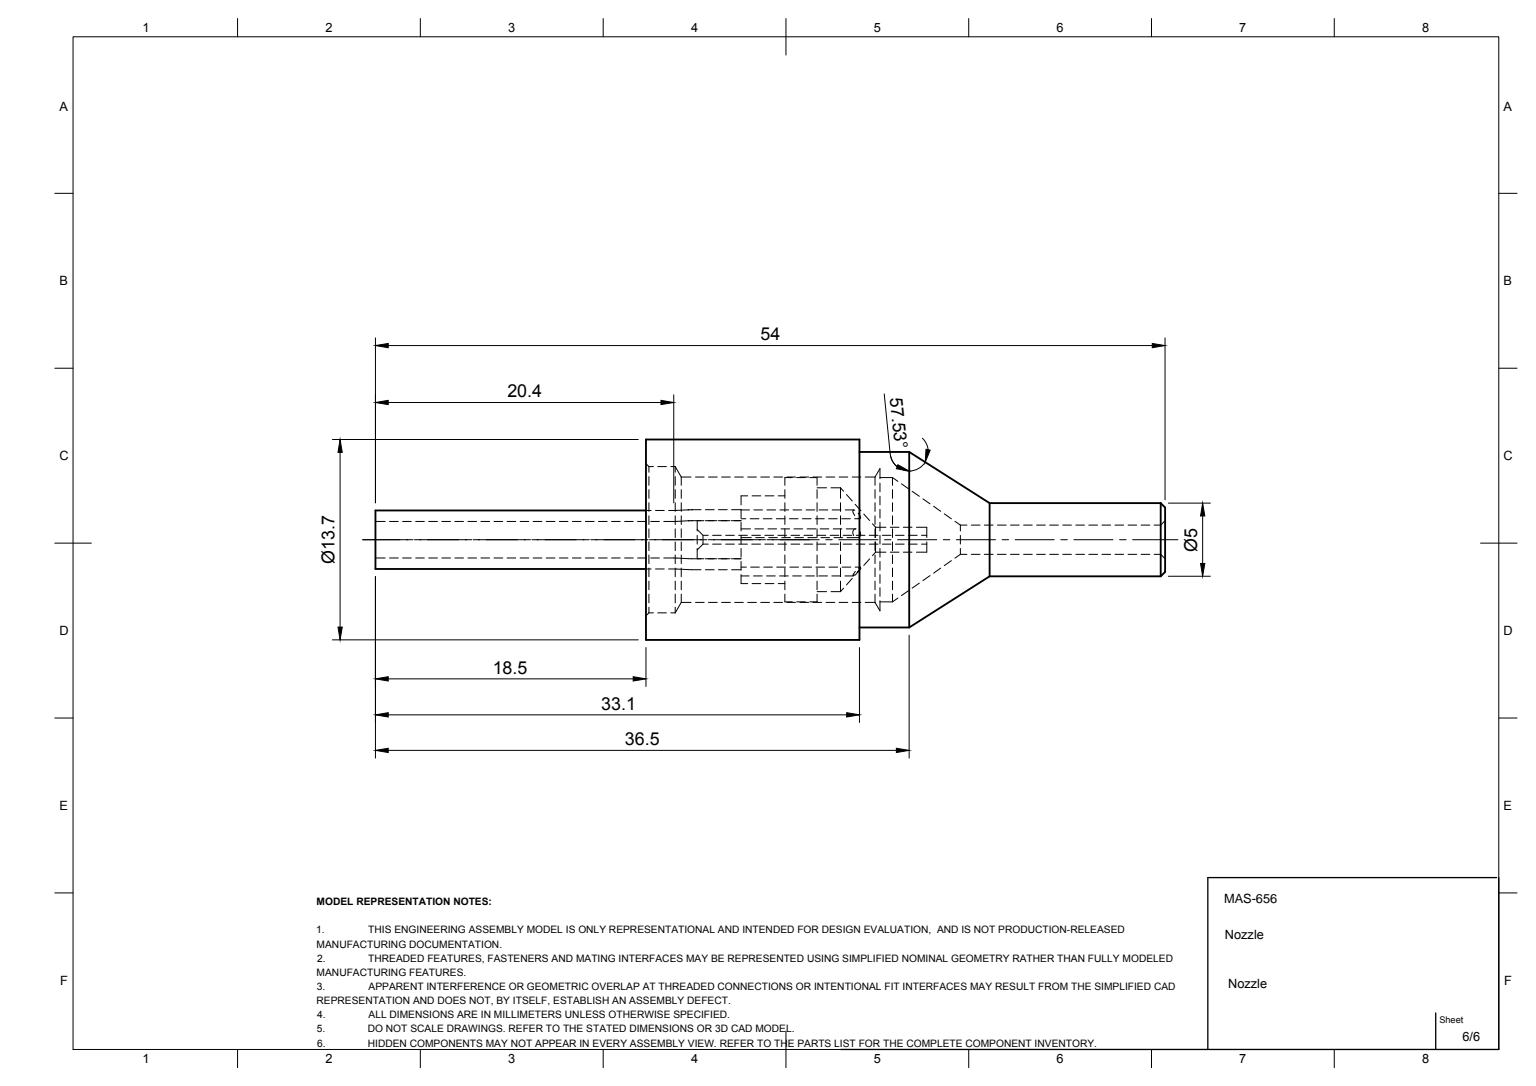
ISO-10303-21;
HEADER;
FILE_DESCRIPTION((''),'2;1');
FILE_NAME('Nozzle.step','2026-10-09T09:41:22-07:00',(''),(''),'','','');
FILE_SCHEMA (('AUTOMOTIVE_DESIGN { 1 0 10303 214 3 1 1 }'));
ENDSEC;
DATA;
#10=MECHANICAL_DESIGN_GEOMETRIC_PRESENTATION_REPRESENTATION('',(#75,#76,#77),#4304);
#55=B_SPLINE_SURFACE_WITH_KNOTS('',5,4,((#3896,#3897,#3898,#3899,#3900),
(#3901,#3902,#3903,#3904,#3905),(#3906,#3907,#3908,#3909,#3910),(#3911,
#3912,#3913,#3914,#3915),(#3916,#3917,#3918,#3919,#3920),(#3921,#3922,#3923,
#3924,#3925),(#3926,#3927,#3928,#3929,#3930),(#3931,#3932,#3933,#3934,#3935),
(#3936,#3937,#3938,#3939,#3940)),.UNSPECIFIED.,.F.,.F.,.F.,(6,3,6),(5,5),
(0.,2.00592385339,5.72401149719),(0.,4.),.UNSPECIFIED.) ;
#56=B_SPLINE_SURFACE_WITH_KNOTS('',5,4,((#4027,#4028,#4029,#4030,#4031),
(#4032,#4033,#4034,#4035,#4036),(#4037,#4038,#4039,#4040,#4041),(#4042,
#4043,#4044,#4045,#4046),(#4047,#4048,#4049,#4050,#4051),(#4052,#4053,#4054,
#4055,#4056),(#4057,#4058,#4059,#4060,#4061),(#4062,#4063,#4064,#4065,#4066),
(#4067,#4068,#4069,#4070,#4071)),.UNSPECIFIED.,.F.,.F.,.F.,(6,3,6),(5,5),
(1.14412490986064,4.56688370431,6.86913676329339),(0.,4.0003840073707),
 .UNSPECIFIED.) ;
#57=B_SPLINE_SURFACE_WITH_KNOTS('',5,4,((#4097,#4098,#4099,#4100,#4101),
(#4102,#4103,#4104,#4105,#4106),(#4107,#4108,#4109,#4110,#4111),(#4112,
#4113,#4114,#4115,#4116),(#4117,#4118,#4119,#4120,#4121),(#4122,#4123,#4124,
#4125,#4126),(#4127,#4128,#4129,#4130,#4131),(#4132,#4133,#4134,#4135,#4136),
(#4137,#4138,#4139,#4140,#4141)),.UNSPECIFIED.,.F.,.F.,.F.,(6,3,6),(5,5),
(1.81018607984298,7.54013629429,10.8709669414987),(-0.00161299974885553,
4.75),.UNSPECIFIED.) ;
#58=B_SPLINE_SURFACE_WITH_KNOTS('',5,4,((#4144,#4145,#4146,#4147,#4148),
(#4149,#4150,#4151,#4152,#4153),(#4154,#4155,#4156,#4157,#4158),(#4159,
#4160,#4161,#4162,#4163),(#4164,#4165,#4166,#4167,#4168),(#4169,#4170,#4171,
#4172,#4173),(#4174,#4175,#4176,#4177,#4178),(#4179,#4180,#4181,#4182,#4183),
(#4184,#4185,#4186,#4187,#4188)),.UNSPECIFIED.,.F.,.F.,.F.,(6,3,6),(5,5),
(-0.00098737241999752,3.59707184609,9.05850997001312),(-0.000987383514799894,
4.75),.UNSPECIFIED.) ;
#59=B_SPLINE_CURVE_WITH_KNOTS('',3,(#3693,#3694,#3695,#3696,#3697,#3698,
#3699,#3700,#3701,#3702,#3703,#3704,#3705,#3706,#3707,#3708,#3709,#3710,
#3711,#3712,#3713,#3714,#3715,#3716,#3717,#3718,#3719,#3720,#3721,#3722,
#3723,#3724,#3725,#3726,#3727,#3728,#3729,#3730),.UNSPECIFIED.,.T.,.F.,
(4,2,2,2,2,2,2,2,2,2,2,2,2,2,2,2,2,2,4),(-0.21266959393403,-0.197090411624007,
-0.181511229313983,-0.168315271544833,-0.161717292660258,-0.155119313775684,
-0.14852133489111,-0.141923356006537,-0.128727398237391,-0.113148215927359,
-0.0975690336173277,-0.0833467314908787,-0.0691244293644297,-0.058954473086547,
-0.0487845168086643,-0.0386145605307833,-0.0284446042529024,-0.0142223021264512,
0.),.UNSPECIFIED.) ;
#60=B_SPLINE_CURVE_WITH_KNOTS('',3,(#3784,#3785,#3786,#3787,#3788,#3789,
#3790,#3791,#3792,#3793,#3794,#3795,#3796,#3797,#3798,#3799,#3800,#3801,
#3802,#3803,#3804,#3805),.UNSPECIFIED.,.F.,.F.,(4,2,2,2,2,2,2,2,2,2,4),
(-0.189267865923668,-0.181511229313965,-0.168315271544809,-0.16171729266023,
-0.155119313775652,-0.148521334891079,-0.141923356006506,-0.128727398237361,
-0.113148215927333,-0.0975690336173056,-0.0836220155565862),
 .UNSPECIFIED.) ;
#61=B_SPLINE_CURVE_WITH_KNOTS('',3,(#3806,#3807,#3808,#3809,#3810,#3811,
#3812,#3813,#3814,#3815,#3816,#3817,#3818,#3819,#3820,#3821,#3822,#3823,
#3824,#3825,#3826,#3827,#3828),.UNSPECIFIED.,.F.,.F.,(4,2,2,2,2,2,2,2,3,
2,4),(-0.0836220155565862,-0.0833467314908613,-0.069124429364417,-0.0589544730865346,
-0.0487845168086522,-0.0386145605307738,-0.0284446042528953,-0.0142223021264476,
0.,0.0155791823100317,0.0234017280103608),.UNSPECIFIED.) ;
#62=B_SPLINE_CURVE_WITH_KNOTS('',3,(#3831,#3832,#3833,#3834,#3835,#3836,
#3837,#3838,#3839,#3840,#3841,#3842,#3843,#3844,#3845,#3846,#3847,#3848,
#3849,#3850,#3851,#3852),.UNSPECIFIED.,.F.,.F.,(4,2,2,2,2,2,2,2,2,2,4),
(-0.189267865923044,-0.181511229313986,-0.16831527154483,-0.161717292660252,
-0.155119313775674,-0.148521334891098,-0.141923356006522,-0.128727398237371,
-0.113148215927341,-0.0975690336173107,-0.083622015556521),
 .UNSPECIFIED.) ;
#63=B_SPLINE_CURVE_WITH_KNOTS('',3,(#3853,#3854,#3855,#3856,#3857,#3858,
#3859,#3860,#3861,#3862,#3863,#3864,#3865,#3866,#3867,#3868,#3869,#3870,
#3871,#3872,#3873,#3874,#3875),.UNSPECIFIED.,.F.,.F.,(4,2,2,2,2,2,2,2,3,
2,4),(-0.083622015556521,-0.0833467314908633,-0.0691244293644159,-0.0589544730865369,
-0.0487845168086579,-0.0386145605307766,-0.0284446042528953,-0.0142223021264477,
0.,0.0155791823100287,0.0234017280109999),.UNSPECIFIED.) ;
#64=B_SPLINE_CURVE_WITH_KNOTS('',3,(#3943,#3944,#3945,#3946,#3947,#3948,
#3949,#3950,#3951,#3952,#3953,#3954,#3955,#3956,#3957,#3958,#3959,#3960,
#3961,#3962,#3963,#3964,#3965,#3966,#3967,#3968,#3969,#3970,#3971,#3972,
#3973,#3974,#3975,#3976,#3977,#3978,#3979,#3980,#3981,#3982,#3983,#3984,
#3985,#3986,#3987,#3988,#3989,#3990,#3991,#3992,#3993,#3994,#3995,#3996,
#3997,#3998,#3999,#4000,#4001,#4002,#4003,#4004,#4005,#4006,#4007,#4008,
#4009,#4010,#4011,#4012,#4013,#4014,#4015,#4016,#4017,#4018,#4019,#4020,
#4021,#4022,#4023,#4024),.UNSPECIFIED.,.F.,.F.,(4,3,3,3,3,3,3,3,3,3,3,3,
3,3,3,3,3,3,3,3,3,3,3,3,3,3,3,4),(0.,0.225460129220956,0.453336599536279,
0.681938236445323,0.91060483211705,1.13866755087004,1.36461264231086,1.58819548811847,
1.8099184881743,2.00592385339,2.22254168431687,2.44222941463765,2.66492844656066,
2.89048514085975,3.12062538022778,3.35076561959582,3.58299027924597,3.81573661936679,
4.04792384057385,4.27908578852667,4.50801790131295,4.57308155019,4.80116409571626,
5.02706122822092,5.25295836072559,5.47141386284307,5.68615166673345,5.72401149719),
 .UNSPECIFIED.) ;
#67=SHAPE_REPRESENTATION_RELATIONSHIP('SRR','None',#4333,#71) ;
#71=ADVANCED_BREP_SHAPE_REPRESENTATION('',(#81,#82,#83),#4302) ;
#75=STYLED_ITEM('',(#4360),#81) ;
#76=STYLED_ITEM('',(#4360),#82) ;
#77=STYLED_ITEM('',(#4361),#83) ;
#81=MANIFOLD_SOLID_BREP('Body1',#2164) ;
#82=MANIFOLD_SOLID_BREP('Body2',#2165) ;
#83=MANIFOLD_SOLID_BREP('Body3',#2166) ;
#98=FACE_BOUND('',#714,.T.) ;
#99=FACE_BOUND('',#716,.T.) ;
#100=FACE_BOUND('',#718,.T.) ;
#101=FACE_BOUND('',#720,.T.) ;
#102=FACE_BOUND('',#724,.T.) ;
#103=FACE_BOUND('',#728,.T.) ;
#104=FACE_BOUND('',#732,.T.) ;
#105=FACE_BOUND('',#735,.T.) ;
#106=FACE_BOUND('',#738,.T.) ;
#107=FACE_BOUND('',#739,.T.) ;
#108=FACE_BOUND('',#740,.T.) ;
#109=FACE_BOUND('',#741,.T.) ;
#110=FACE_BOUND('',#743,.T.) ;
#111=FACE_BOUND('',#744,.T.) ;
#112=FACE_BOUND('',#745,.T.) ;
#113=FACE_BOUND('',#749,.T.) ;
#114=FACE_BOUND('',#751,.T.) ;
#148=PLANE('',#2399) ;
#149=PLANE('',#2400) ;
#150=PLANE('',#2401) ;
#151=PLANE('',#2402) ;
#152=PLANE('',#2408) ;
#153=PLANE('',#2414) ;
#154=PLANE('',#2421) ;
#155=PLANE('',#2425) ;
#156=PLANE('',#2429) ;
#157=PLANE('',#2435) ;
#158=PLANE('',#2438) ;
#169=TOROIDAL_SURFACE('',#2450,6.00000000000046,4.0000000000003) ;
#170=TOROIDAL_SURFACE('',#2466,6.00000000000046,4.75000000000036) ;
#198=CYLINDRICAL_SURFACE('',#2367,6.85000000000052) ;
#199=CYLINDRICAL_SURFACE('',#2370,6.00000000000046) ;
#200=CYLINDRICAL_SURFACE('',#2375,2.50000000000019) ;
#201=CYLINDRICAL_SURFACE('',#2382,1.00000000000008) ;
#202=CYLINDRICAL_SURFACE('',#2386,4.25000000000032) ;
#203=CYLINDRICAL_SURFACE('',#2391,4.28300000000033) ;
#204=CYLINDRICAL_SURFACE('',#2395,5.00000000000038) ;
#205=CYLINDRICAL_SURFACE('',#2403,0.300000000000023) ;
#206=CYLINDRICAL_SURFACE('',#2405,1.3000000000001) ;
#207=CYLINDRICAL_SURFACE('',#2412,0.300000000000023) ;
#208=CYLINDRICAL_SURFACE('',#2416,0.850000000000065) ;
#209=CYLINDRICAL_SURFACE('',#2418,3.55000000000027) ;
#210=CYLINDRICAL_SURFACE('',#2423,4.25000000000032) ;
#211=CYLINDRICAL_SURFACE('',#2427,3.00000000000023) ;
#212=CYLINDRICAL_SURFACE('',#2433,0.300000000000023) ;
#213=CYLINDRICAL_SURFACE('',#2434,0.300000000000023) ;
#214=CYLINDRICAL_SURFACE('',#2441,1.3000000000001) ;
#215=CYLINDRICAL_SURFACE('',#2447,2.00000000000015) ;
#216=CYLINDRICAL_SURFACE('',#2454,2.05000000000016) ;
#217=CYLINDRICAL_SURFACE('',#2462,1.2500000000001) ;
#303=LINE('',#3624,#422) ;
#304=LINE('',#3630,#423) ;
#305=LINE('',#3634,#424) ;
#306=LINE('',#3639,#425) ;
#307=LINE('',#3642,#426) ;
#308=LINE('',#3648,#427) ;
#309=LINE('',#3653,#428) ;
#310=LINE('',#3656,#429) ;
#311=LINE('',#3661,#430) ;
#312=LINE('',#3666,#431) ;
#313=LINE('',#3671,#432) ;
#314=LINE('',#3674,#433) ;
#315=LINE('',#3679,#434) ;
#316=LINE('',#3682,#435) ;
#317=LINE('',#3692,#436) ;
#318=LINE('',#3735,#437) ;
#319=LINE('',#3743,#438) ;
#320=LINE('',#3746,#439) ;
#321=LINE('',#3753,#440) ;
#322=LINE('',#3759,#441) ;
#323=LINE('',#3766,#442) ;
#324=LINE('',#3773,#443) ;
#325=LINE('',#3781,#444) ;
#326=LINE('',#3877,#445) ;
#327=LINE('',#3879,#446) ;
#328=LINE('',#3895,#447) ;
#329=LINE('',#4077,#448) ;
#330=LINE('',#4087,#449) ;
#331=LINE('',#4096,#450) ;
#332=LINE('',#4191,#451) ;
#333=LINE('',#4196,#452) ;
#422=VECTOR('',#2922,6.85000000000052) ;
#423=VECTOR('',#2929,6.00000000000046) ;
#424=VECTOR('',#2934,2.50000000000019) ;
#425=VECTOR('',#2941,2.50000000000019) ;
#426=VECTOR('',#2944,2.20000000000017) ;
#427=VECTOR('',#2951,1.00000000000008) ;
#428=VECTOR('',#2958,1.00000000000008) ;
#429=VECTOR('',#2961,1.00000000000008) ;
#430=VECTOR('',#2968,4.25000000000032) ;
#431=VECTOR('',#2973,4.28300000000033) ;
#432=VECTOR('',#2980,4.28300000000033) ;
#433=VECTOR('',#2983,4.28300000000033) ;
#434=VECTOR('',#2990,5.00000000000038) ;
#435=VECTOR('',#2993,5.00000000000038) ;
#436=VECTOR('',#3008,0.300000000000023) ;
#437=VECTOR('',#3013,1.3000000000001) ;
#438=VECTOR('',#3024,0.300000000000023) ;
#439=VECTOR('',#3027,0.300000000000023) ;
#440=VECTOR('',#3036,0.850000000000065) ;
#441=VECTOR('',#3043,3.55000000000027) ;
#442=VECTOR('',#3052,4.25000000000032) ;
#443=VECTOR('',#3061,3.00000000000023) ;
#444=VECTOR('',#3072,0.850000000000065) ;
#445=VECTOR('',#3075,0.300000000000023) ;
#446=VECTOR('',#3078,0.300000000000023) ;
#447=VECTOR('',#3097,1.3000000000001) ;
#448=VECTOR('',#3108,2.00000000000015) ;
#449=VECTOR('',#3121,2.05000000000016) ;
#450=VECTOR('',#3132,2.00000000000015) ;
#451=VECTOR('',#3139,1.2500000000001) ;
#452=VECTOR('',#3146,1.2500000000001) ;
#466=CONICAL_SURFACE('',#2373,2.50000000000019,0.566729217524) ;
#467=CONICAL_SURFACE('',#2377,2.20000000000017,0.785398163397) ;
#468=CONICAL_SURFACE('',#2379,1.00000000000008,0.785398163397) ;
#469=CONICAL_SURFACE('',#2384,1.00000000000008,0.610865238198) ;
#470=CONICAL_SURFACE('',#2388,4.28300000000033,1.0471975512) ;
#471=CONICAL_SURFACE('',#2393,4.28300000000033,1.0471975512) ;
#472=CONICAL_SURFACE('',#2397,5.00000000000038,0.785398163397) ;
#473=CONICAL_SURFACE('',#2410,0.300000000000023,0.785398163397) ;
#474=CONICAL_SURFACE('',#2432,0.850000000000065,0.844153986113) ;
#475=CONICAL_SURFACE('',#2457,2.00000000000015,0.0499583957219) ;
#476=CONICAL_SURFACE('',#2464,1.2500000000001,0.0499583957219) ;
#550=FACE_OUTER_BOUND('',#699,.T.) ;
#551=FACE_OUTER_BOUND('',#700,.T.) ;
#552=FACE_OUTER_BOUND('',#701,.T.) ;
#553=FACE_OUTER_BOUND('',#702,.T.) ;
#554=FACE_OUTER_BOUND('',#703,.T.) ;
#555=FACE_OUTER_BOUND('',#704,.T.) ;
#556=FACE_OUTER_BOUND('',#705,.T.) ;
#557=FACE_OUTER_BOUND('',#706,.T.) ;
#558=FACE_OUTER_BOUND('',#707,.T.) ;
#559=FACE_OUTER_BOUND('',#708,.T.) ;
#560=FACE_OUTER_BOUND('',#709,.T.) ;
#561=FACE_OUTER_BOUND('',#710,.T.) ;
#562=FACE_OUTER_BOUND('',#711,.T.) ;
#563=FACE_OUTER_BOUND('',#712,.T.) ;
#564=FACE_OUTER_BOUND('',#713,.T.) ;
#565=FACE_OUTER_BOUND('',#715,.T.) ;
#566=FACE_OUTER_BOUND('',#717,.T.) ;
#567=FACE_OUTER_BOUND('',#719,.T.) ;
#568=FACE_OUTER_BOUND('',#721,.T.) ;
#569=FACE_OUTER_BOUND('',#722,.T.) ;
#570=FACE_OUTER_BOUND('',#723,.T.) ;
#571=FACE_OUTER_BOUND('',#725,.T.) ;
#572=FACE_OUTER_BOUND('',#726,.T.) ;
#573=FACE_OUTER_BOUND('',#727,.T.) ;
#574=FACE_OUTER_BOUND('',#729,.T.) ;
#575=FACE_OUTER_BOUND('',#730,.T.) ;
#576=FACE_OUTER_BOUND('',#731,.T.) ;
#577=FACE_OUTER_BOUND('',#733,.T.) ;
#578=FACE_OUTER_BOUND('',#734,.T.) ;
#579=FACE_OUTER_BOUND('',#736,.T.) ;
#580=FACE_OUTER_BOUND('',#737,.T.) ;
#581=FACE_OUTER_BOUND('',#742,.T.) ;
#582=FACE_OUTER_BOUND('',#746,.T.) ;
#583=FACE_OUTER_BOUND('',#747,.T.) ;
#584=FACE_OUTER_BOUND('',#748,.T.) ;
#585=FACE_OUTER_BOUND('',#750,.T.) ;
#586=FACE_OUTER_BOUND('',#752,.T.) ;
#587=FACE_OUTER_BOUND('',#753,.T.) ;
#588=FACE_OUTER_BOUND('',#754,.T.) ;
#589=FACE_OUTER_BOUND('',#755,.T.) ;
#590=FACE_OUTER_BOUND('',#756,.T.) ;
#591=FACE_OUTER_BOUND('',#757,.T.) ;
#592=FACE_OUTER_BOUND('',#758,.T.) ;
#593=FACE_OUTER_BOUND('',#759,.T.) ;
#594=FACE_OUTER_BOUND('',#760,.T.) ;
#595=FACE_OUTER_BOUND('',#761,.T.) ;
#596=FACE_OUTER_BOUND('',#762,.T.) ;
#597=FACE_OUTER_BOUND('',#763,.T.) ;
#699=EDGE_LOOP('',(#1751,#1752,#1753,#1754)) ;
#700=EDGE_LOOP('',(#1755,#1756,#1757,#1758)) ;
#701=EDGE_LOOP('',(#1759,#1760,#1761,#1762)) ;
#702=EDGE_LOOP('',(#1763,#1764,#1765,#1766)) ;
#703=EDGE_LOOP('',(#1767,#1768,#1769,#1770)) ;
#704=EDGE_LOOP('',(#1771,#1772,#1773,#1774)) ;
#705=EDGE_LOOP('',(#1775,#1776,#1777,#1778)) ;
#706=EDGE_LOOP('',(#1779,#1780,#1781,#1782)) ;
#707=EDGE_LOOP('',(#1783,#1784,#1785,#1786)) ;
#708=EDGE_LOOP('',(#1787,#1788,#1789,#1790)) ;
#709=EDGE_LOOP('',(#1791,#1792,#1793,#1794)) ;
#710=EDGE_LOOP('',(#1795,#1796,#1797,#1798)) ;
#711=EDGE_LOOP('',(#1799,#1800,#1801,#1802)) ;
#712=EDGE_LOOP('',(#1803,#1804,#1805,#1806)) ;
#713=EDGE_LOOP('',(#1807)) ;
#714=EDGE_LOOP('',(#1808)) ;
#715=EDGE_LOOP('',(#1809)) ;
#716=EDGE_LOOP('',(#1810)) ;
#717=EDGE_LOOP('',(#1811)) ;
#718=EDGE_LOOP('',(#1812)) ;
#719=EDGE_LOOP('',(#1813)) ;
#720=EDGE_LOOP('',(#1814)) ;
#721=EDGE_LOOP('',(#1815,#1816,#1817,#1818)) ;
#722=EDGE_LOOP('',(#1819,#1820,#1821,#1822)) ;
#723=EDGE_LOOP('',(#1823)) ;
#724=EDGE_LOOP('',(#1824)) ;
#725=EDGE_LOOP('',(#1825,#1826,#1827,#1828)) ;
#726=EDGE_LOOP('',(#1829,#1830,#1831,#1832)) ;
#727=EDGE_LOOP('',(#1833)) ;
#728=EDGE_LOOP('',(#1834)) ;
#729=EDGE_LOOP('',(#1835,#1836,#1837,#1838)) ;
#730=EDGE_LOOP('',(#1839,#1840,#1841,#1842)) ;
#731=EDGE_LOOP('',(#1843)) ;
#732=EDGE_LOOP('',(#1844)) ;
#733=EDGE_LOOP('',(#1845,#1846,#1847,#1848)) ;
#734=EDGE_LOOP('',(#1849)) ;
#735=EDGE_LOOP('',(#1850)) ;
#736=EDGE_LOOP('',(#1851,#1852,#1853,#1854)) ;
#737=EDGE_LOOP('',(#1855)) ;
#738=EDGE_LOOP('',(#1856)) ;
#739=EDGE_LOOP('',(#1857)) ;
#740=EDGE_LOOP('',(#1858)) ;
#741=EDGE_LOOP('',(#1859)) ;
#742=EDGE_LOOP('',(#1860,#1861,#1862,#1863)) ;
#743=EDGE_LOOP('',(#1864,#1865)) ;
#744=EDGE_LOOP('',(#1866,#1867)) ;
#745=EDGE_LOOP('',(#1868)) ;
#746=EDGE_LOOP('',(#1869,#1870,#1871,#1872,#1873)) ;
#747=EDGE_LOOP('',(#1874,#1875,#1876,#1877,#1878)) ;
#748=EDGE_LOOP('',(#1879)) ;
#749=EDGE_LOOP('',(#1880)) ;
#750=EDGE_LOOP('',(#1881)) ;
#751=EDGE_LOOP('',(#1882)) ;
#752=EDGE_LOOP('',(#1883,#1884,#1885,#1886,#1887)) ;
#753=EDGE_LOOP('',(#1888,#1889,#1890,#1891)) ;
#754=EDGE_LOOP('',(#1892,#1893,#1894,#1895)) ;
#755=EDGE_LOOP('',(#1896,#1897,#1898,#1899,#1900)) ;
#756=EDGE_LOOP('',(#1901,#1902,#1903,#1904,#1905,#1906)) ;
#757=EDGE_LOOP('',(#1907,#1908,#1909,#1910,#1911)) ;
#758=EDGE_LOOP('',(#1912,#1913,#1914,#1915,#1916,#1917)) ;
#759=EDGE_LOOP('',(#1918,#1919,#1920,#1921)) ;
#760=EDGE_LOOP('',(#1922,#1923,#1924,#1925)) ;
#761=EDGE_LOOP('',(#1926,#1927,#1928,#1929)) ;
#762=EDGE_LOOP('',(#1930,#1931,#1932,#1933,#1934)) ;
#763=EDGE_LOOP('',(#1935,#1936,#1937,#1938)) ;
#864=CIRCLE('',#2368,6.85000000000052) ;
#865=CIRCLE('',#2369,6.85000000000052) ;
#866=CIRCLE('',#2371,6.00000000000046) ;
#867=CIRCLE('',#2372,6.00000000000046) ;
#868=CIRCLE('',#2374,2.50000000000019) ;
#869=CIRCLE('',#2376,2.50000000000019) ;
#870=CIRCLE('',#2378,2.20000000000017) ;
#871=CIRCLE('',#2380,1.00000000000008) ;
#872=CIRCLE('',#2381,1.3000000000001) ;
#873=CIRCLE('',#2383,1.00000000000008) ;
#874=CIRCLE('',#2385,4.25000000000032) ;
#875=CIRCLE('',#2387,4.25000000000032) ;
#876=CIRCLE('',#2389,4.28300000000033) ;
#877=CIRCLE('',#2390,4.86400000000037) ;
#878=CIRCLE('',#2392,4.28300000000033) ;
#879=CIRCLE('',#2394,5.00000000000038) ;
#880=CIRCLE('',#2396,5.00000000000038) ;
#881=CIRCLE('',#2398,5.20000000000039) ;
#882=CIRCLE('',#2404,0.300000000000023) ;
#883=CIRCLE('',#2406,1.3000000000001) ;
#884=CIRCLE('',#2407,1.3000000000001) ;
#885=CIRCLE('',#2409,0.700000000000053) ;
#886=CIRCLE('',#2411,0.300000000000023) ;
#887=CIRCLE('',#2413,0.300000000000023) ;
#888=CIRCLE('',#2415,0.850000000000065) ;
#889=CIRCLE('',#2417,0.850000000000065) ;
#890=CIRCLE('',#2419,3.55000000000027) ;
#891=CIRCLE('',#2420,3.55000000000027) ;
#892=CIRCLE('',#2422,4.25000000000032) ;
#893=CIRCLE('',#2424,4.25000000000032) ;
#894=CIRCLE('',#2426,3.00000000000023) ;
#895=CIRCLE('',#2428,3.00000000000023) ;
#896=CIRCLE('',#2430,0.300000000000023) ;
#897=CIRCLE('',#2431,0.300000000000023) ;
#898=CIRCLE('',#2436,2.00000000000015) ;
#899=CIRCLE('',#2437,1.2500000000001) ;
#900=CIRCLE('',#2439,2.05000000000016) ;
#901=CIRCLE('',#2440,1.3000000000001) ;
#902=CIRCLE('',#2442,1.3000000000001) ;
#903=CIRCLE('',#2443,1.3000000000001) ;
#904=CIRCLE('',#2444,4.00000013651843) ;
#905=CIRCLE('',#2445,3.9999999789986) ;
#906=CIRCLE('',#2446,1.29500935558696) ;
#907=CIRCLE('',#2448,2.00000000000015) ;
#908=CIRCLE('',#2449,2.00000000000015) ;
#909=CIRCLE('',#2451,2.00499064449015) ;
#910=CIRCLE('',#2452,4.0000000000003) ;
#911=CIRCLE('',#2453,2.00499064449015) ;
#912=CIRCLE('',#2455,2.05000000000016) ;
#913=CIRCLE('',#2456,2.05000000000016) ;
#914=CIRCLE('',#2458,2.04407360967015) ;
#915=CIRCLE('',#2459,2.04407360967015) ;
#916=CIRCLE('',#2460,4.75024664381333) ;
#917=CIRCLE('',#2461,4.74999996695025) ;
#918=CIRCLE('',#2463,1.2500000000001) ;
#919=CIRCLE('',#2465,1.2559263903301) ;
#920=CIRCLE('',#2467,4.75000000000036) ;
#1056=VERTEX_POINT('',#3621) ;
#1057=VERTEX_POINT('',#3623) ;
#1058=VERTEX_POINT('',#3627) ;
#1059=VERTEX_POINT('',#3629) ;
#1060=VERTEX_POINT('',#3633) ;
#1061=VERTEX_POINT('',#3637) ;
#1062=VERTEX_POINT('',#3641) ;
#1063=VERTEX_POINT('',#3645) ;
#1064=VERTEX_POINT('',#3647) ;
#1065=VERTEX_POINT('',#3651) ;
#1066=VERTEX_POINT('',#3655) ;
#1067=VERTEX_POINT('',#3659) ;
#1068=VERTEX_POINT('',#3663) ;
#1069=VERTEX_POINT('',#3665) ;
#1070=VERTEX_POINT('',#3669) ;
#1071=VERTEX_POINT('',#3673) ;
#1072=VERTEX_POINT('',#3677) ;
#1073=VERTEX_POINT('',#3681) ;
#1074=VERTEX_POINT('',#3689) ;
#1075=VERTEX_POINT('',#3691) ;
#1076=VERTEX_POINT('',#3732) ;
#1077=VERTEX_POINT('',#3734) ;
#1078=VERTEX_POINT('',#3738) ;
#1079=VERTEX_POINT('',#3741) ;
#1080=VERTEX_POINT('',#3745) ;
#1081=VERTEX_POINT('',#3749) ;
#1082=VERTEX_POINT('',#3752) ;
#1083=VERTEX_POINT('',#3756) ;
#1084=VERTEX_POINT('',#3758) ;
#1085=VERTEX_POINT('',#3762) ;
#1086=VERTEX_POINT('',#3765) ;
#1087=VERTEX_POINT('',#3769) ;
#1088=VERTEX_POINT('',#3772) ;
#1089=VERTEX_POINT('',#3776) ;
#1090=VERTEX_POINT('',#3778) ;
#1091=VERTEX_POINT('',#3782) ;
#1092=VERTEX_POINT('',#3783) ;
#1093=VERTEX_POINT('',#3829) ;
#1094=VERTEX_POINT('',#3830) ;
#1095=VERTEX_POINT('',#3881) ;
#1096=VERTEX_POINT('',#3883) ;
#1097=VERTEX_POINT('',#3886) ;
#1098=VERTEX_POINT('',#3888) ;
#1099=VERTEX_POINT('',#3891) ;
#1100=VERTEX_POINT('',#3892) ;
#1101=VERTEX_POINT('',#3941) ;
#1102=VERTEX_POINT('',#3942) ;
#1103=VERTEX_POINT('',#4074) ;
#1104=VERTEX_POINT('',#4075) ;
#1105=VERTEX_POINT('',#4080) ;
#1106=VERTEX_POINT('',#4081) ;
#1107=VERTEX_POINT('',#4086) ;
#1108=VERTEX_POINT('',#4088) ;
#1109=VERTEX_POINT('',#4092) ;
#1110=VERTEX_POINT('',#4093) ;
#1111=VERTEX_POINT('',#4190) ;
#1112=VERTEX_POINT('',#4194) ;
#1297=EDGE_CURVE('',#1056,#1056,#864,.T.) ;
#1298=EDGE_CURVE('',#1056,#1057,#303,.T.) ;
#1299=EDGE_CURVE('',#1057,#1057,#865,.T.) ;
#1300=EDGE_CURVE('',#1058,#1058,#866,.T.) ;
#1301=EDGE_CURVE('',#1058,#1059,#304,.T.) ;
#1302=EDGE_CURVE('',#1059,#1059,#867,.T.) ;
#1303=EDGE_CURVE('',#1058,#1060,#305,.T.) ;
#1304=EDGE_CURVE('',#1060,#1060,#868,.F.) ;
#1305=EDGE_CURVE('',#1061,#1061,#869,.T.) ;
#1306=EDGE_CURVE('',#1061,#1060,#306,.T.) ;
#1307=EDGE_CURVE('',#1061,#1062,#307,.T.) ;
#1308=EDGE_CURVE('',#1062,#1062,#870,.F.) ;
#1309=EDGE_CURVE('',#1063,#1063,#871,.T.) ;
#1310=EDGE_CURVE('',#1063,#1064,#308,.T.) ;
#1311=EDGE_CURVE('',#1064,#1064,#872,.T.) ;
#1312=EDGE_CURVE('',#1065,#1065,#873,.T.) ;
#1313=EDGE_CURVE('',#1065,#1063,#309,.T.) ;
#1314=EDGE_CURVE('',#1065,#1066,#310,.T.) ;
#1315=EDGE_CURVE('',#1066,#1066,#874,.F.) ;
#1316=EDGE_CURVE('',#1067,#1067,#875,.T.) ;
#1317=EDGE_CURVE('',#1067,#1066,#311,.T.) ;
#1318=EDGE_CURVE('',#1068,#1068,#876,.T.) ;
#1319=EDGE_CURVE('',#1068,#1069,#312,.T.) ;
#1320=EDGE_CURVE('',#1069,#1069,#877,.T.) ;
#1321=EDGE_CURVE('',#1070,#1070,#878,.T.) ;
#1322=EDGE_CURVE('',#1070,#1068,#313,.T.) ;
#1323=EDGE_CURVE('',#1070,#1071,#314,.T.) ;
#1324=EDGE_CURVE('',#1071,#1071,#879,.F.) ;
#1325=EDGE_CURVE('',#1072,#1072,#880,.T.) ;
#1326=EDGE_CURVE('',#1072,#1071,#315,.T.) ;
#1327=EDGE_CURVE('',#1072,#1073,#316,.T.) ;
#1328=EDGE_CURVE('',#1073,#1073,#881,.F.) ;
#1329=EDGE_CURVE('',#1074,#1074,#882,.T.) ;
#1330=EDGE_CURVE('',#1074,#1075,#317,.T.) ;
#1331=EDGE_CURVE('',#1075,#1075,#59,.T.) ;
#1332=EDGE_CURVE('',#1076,#1076,#883,.T.) ;
#1333=EDGE_CURVE('',#1076,#1077,#318,.T.) ;
#1334=EDGE_CURVE('',#1077,#1077,#884,.T.) ;
#1335=EDGE_CURVE('',#1078,#1078,#885,.T.) ;
#1336=EDGE_CURVE('',#1079,#1079,#886,.F.) ;
#1337=EDGE_CURVE('',#1079,#1078,#319,.T.) ;
#1338=EDGE_CURVE('',#1079,#1080,#320,.T.) ;
#1339=EDGE_CURVE('',#1080,#1080,#887,.T.) ;
#1340=EDGE_CURVE('',#1081,#1081,#888,.T.) ;
#1341=EDGE_CURVE('',#1081,#1082,#321,.T.) ;
#1342=EDGE_CURVE('',#1082,#1082,#889,.T.) ;
#1343=EDGE_CURVE('',#1083,#1083,#890,.T.) ;
#1344=EDGE_CURVE('',#1083,#1084,#322,.T.) ;
#1345=EDGE_CURVE('',#1084,#1084,#891,.T.) ;
#1346=EDGE_CURVE('',#1085,#1085,#892,.T.) ;
#1347=EDGE_CURVE('',#1085,#1086,#323,.T.) ;
#1348=EDGE_CURVE('',#1086,#1086,#893,.T.) ;
#1349=EDGE_CURVE('',#1087,#1087,#894,.T.) ;
#1350=EDGE_CURVE('',#1087,#1088,#324,.T.) ;
#1351=EDGE_CURVE('',#1088,#1088,#895,.T.) ;
#1352=EDGE_CURVE('',#1089,#1089,#896,.T.) ;
#1353=EDGE_CURVE('',#1090,#1090,#897,.T.) ;
#1354=EDGE_CURVE('',#1083,#1082,#325,.T.) ;
#1355=EDGE_CURVE('',#1091,#1092,#60,.T.) ;
#1356=EDGE_CURVE('',#1092,#1091,#61,.T.) ;
#1357=EDGE_CURVE('',#1093,#1094,#62,.T.) ;
#1358=EDGE_CURVE('',#1094,#1093,#63,.T.) ;
#1359=EDGE_CURVE('',#1089,#1092,#326,.T.) ;
#1360=EDGE_CURVE('',#1090,#1094,#327,.T.) ;
#1361=EDGE_CURVE('',#1095,#1095,#898,.T.) ;
#1362=EDGE_CURVE('',#1096,#1096,#899,.T.) ;
#1363=EDGE_CURVE('',#1097,#1097,#900,.T.) ;
#1364=EDGE_CURVE('',#1098,#1098,#901,.T.) ;
#1365=EDGE_CURVE('',#1099,#1100,#902,.F.) ;
#1366=EDGE_CURVE('',#1100,#1099,#903,.F.) ;
#1367=EDGE_CURVE('',#1099,#1098,#328,.T.) ;
#1368=EDGE_CURVE('',#1101,#1102,#64,.T.) ;
#1369=EDGE_CURVE('',#1102,#1099,#904,.F.) ;
#1370=EDGE_CURVE('',#1101,#1100,#905,.F.) ;
#1371=EDGE_CURVE('',#1102,#1101,#906,.T.) ;
#1372=EDGE_CURVE('',#1103,#1104,#907,.F.) ;
#1373=EDGE_CURVE('',#1104,#1095,#329,.T.) ;
#1374=EDGE_CURVE('',#1104,#1103,#908,.F.) ;
#1375=EDGE_CURVE('',#1105,#1106,#909,.F.) ;
#1376=EDGE_CURVE('',#1106,#1103,#910,.T.) ;
#1377=EDGE_CURVE('',#1106,#1105,#911,.F.) ;
#1378=EDGE_CURVE('',#1097,#1107,#330,.T.) ;
#1379=EDGE_CURVE('',#1107,#1108,#912,.T.) ;
#1380=EDGE_CURVE('',#1108,#1107,#913,.T.) ;
#1381=EDGE_CURVE('',#1109,#1110,#914,.T.) ;
#1382=EDGE_CURVE('',#1110,#1109,#915,.T.) ;
#1383=EDGE_CURVE('',#1110,#1105,#331,.T.) ;
#1384=EDGE_CURVE('',#1107,#1110,#916,.F.) ;
#1385=EDGE_CURVE('',#1108,#1109,#917,.F.) ;
#1386=EDGE_CURVE('',#1096,#1111,#332,.T.) ;
#1387=EDGE_CURVE('',#1111,#1111,#918,.T.) ;
#1388=EDGE_CURVE('',#1112,#1112,#919,.T.) ;
#1389=EDGE_CURVE('',#1112,#1102,#333,.T.) ;
#1390=EDGE_CURVE('',#1112,#1111,#920,.T.) ;
#1751=ORIENTED_EDGE('',*,*,#1297,.F.) ;
#1752=ORIENTED_EDGE('',*,*,#1298,.T.) ;
#1753=ORIENTED_EDGE('',*,*,#1299,.T.) ;
#1754=ORIENTED_EDGE('',*,*,#1298,.F.) ;
#1755=ORIENTED_EDGE('',*,*,#1300,.F.) ;
#1756=ORIENTED_EDGE('',*,*,#1301,.T.) ;
#1757=ORIENTED_EDGE('',*,*,#1302,.T.) ;
#1758=ORIENTED_EDGE('',*,*,#1301,.F.) ;
#1759=ORIENTED_EDGE('',*,*,#1300,.T.) ;
#1760=ORIENTED_EDGE('',*,*,#1303,.T.) ;
#1761=ORIENTED_EDGE('',*,*,#1304,.F.) ;
#1762=ORIENTED_EDGE('',*,*,#1303,.F.) ;
#1763=ORIENTED_EDGE('',*,*,#1305,.F.) ;
#1764=ORIENTED_EDGE('',*,*,#1306,.T.) ;
#1765=ORIENTED_EDGE('',*,*,#1304,.T.) ;
#1766=ORIENTED_EDGE('',*,*,#1306,.F.) ;
#1767=ORIENTED_EDGE('',*,*,#1305,.T.) ;
#1768=ORIENTED_EDGE('',*,*,#1307,.T.) ;
#1769=ORIENTED_EDGE('',*,*,#1308,.F.) ;
#1770=ORIENTED_EDGE('',*,*,#1307,.F.) ;
#1771=ORIENTED_EDGE('',*,*,#1309,.F.) ;
#1772=ORIENTED_EDGE('',*,*,#1310,.T.) ;
#1773=ORIENTED_EDGE('',*,*,#1311,.T.) ;
#1774=ORIENTED_EDGE('',*,*,#1310,.F.) ;
#1775=ORIENTED_EDGE('',*,*,#1312,.F.) ;
#1776=ORIENTED_EDGE('',*,*,#1313,.T.) ;
#1777=ORIENTED_EDGE('',*,*,#1309,.T.) ;
#1778=ORIENTED_EDGE('',*,*,#1313,.F.) ;
#1779=ORIENTED_EDGE('',*,*,#1312,.T.) ;
#1780=ORIENTED_EDGE('',*,*,#1314,.T.) ;
#1781=ORIENTED_EDGE('',*,*,#1315,.F.) ;
#1782=ORIENTED_EDGE('',*,*,#1314,.F.) ;
#1783=ORIENTED_EDGE('',*,*,#1316,.F.) ;
#1784=ORIENTED_EDGE('',*,*,#1317,.T.) ;
#1785=ORIENTED_EDGE('',*,*,#1315,.T.) ;
#1786=ORIENTED_EDGE('',*,*,#1317,.F.) ;
#1787=ORIENTED_EDGE('',*,*,#1318,.F.) ;
#1788=ORIENTED_EDGE('',*,*,#1319,.T.) ;
#1789=ORIENTED_EDGE('',*,*,#1320,.T.) ;
#1790=ORIENTED_EDGE('',*,*,#1319,.F.) ;
#1791=ORIENTED_EDGE('',*,*,#1321,.F.) ;
#1792=ORIENTED_EDGE('',*,*,#1322,.T.) ;
#1793=ORIENTED_EDGE('',*,*,#1318,.T.) ;
#1794=ORIENTED_EDGE('',*,*,#1322,.F.) ;
#1795=ORIENTED_EDGE('',*,*,#1321,.T.) ;
#1796=ORIENTED_EDGE('',*,*,#1323,.T.) ;
#1797=ORIENTED_EDGE('',*,*,#1324,.F.) ;
#1798=ORIENTED_EDGE('',*,*,#1323,.F.) ;
#1799=ORIENTED_EDGE('',*,*,#1325,.F.) ;
#1800=ORIENTED_EDGE('',*,*,#1326,.T.) ;
#1801=ORIENTED_EDGE('',*,*,#1324,.T.) ;
#1802=ORIENTED_EDGE('',*,*,#1326,.F.) ;
#1803=ORIENTED_EDGE('',*,*,#1325,.T.) ;
#1804=ORIENTED_EDGE('',*,*,#1327,.T.) ;
#1805=ORIENTED_EDGE('',*,*,#1328,.F.) ;
#1806=ORIENTED_EDGE('',*,*,#1327,.F.) ;
#1807=ORIENTED_EDGE('',*,*,#1297,.T.) ;
#1808=ORIENTED_EDGE('',*,*,#1302,.F.) ;
#1809=ORIENTED_EDGE('',*,*,#1308,.T.) ;
#1810=ORIENTED_EDGE('',*,*,#1311,.F.) ;
#1811=ORIENTED_EDGE('',*,*,#1320,.F.) ;
#1812=ORIENTED_EDGE('',*,*,#1316,.T.) ;
#1813=ORIENTED_EDGE('',*,*,#1299,.F.) ;
#1814=ORIENTED_EDGE('',*,*,#1328,.T.) ;
#1815=ORIENTED_EDGE('',*,*,#1329,.F.) ;
#1816=ORIENTED_EDGE('',*,*,#1330,.T.) ;
#1817=ORIENTED_EDGE('',*,*,#1331,.T.) ;
#1818=ORIENTED_EDGE('',*,*,#1330,.F.) ;
#1819=ORIENTED_EDGE('',*,*,#1332,.F.) ;
#1820=ORIENTED_EDGE('',*,*,#1333,.T.) ;
#1821=ORIENTED_EDGE('',*,*,#1334,.T.) ;
#1822=ORIENTED_EDGE('',*,*,#1333,.F.) ;
#1823=ORIENTED_EDGE('',*,*,#1334,.F.) ;
#1824=ORIENTED_EDGE('',*,*,#1335,.T.) ;
#1825=ORIENTED_EDGE('',*,*,#1336,.T.) ;
#1826=ORIENTED_EDGE('',*,*,#1337,.T.) ;
#1827=ORIENTED_EDGE('',*,*,#1335,.F.) ;
#1828=ORIENTED_EDGE('',*,*,#1337,.F.) ;
#1829=ORIENTED_EDGE('',*,*,#1336,.F.) ;
#1830=ORIENTED_EDGE('',*,*,#1338,.T.) ;
#1831=ORIENTED_EDGE('',*,*,#1339,.T.) ;
#1832=ORIENTED_EDGE('',*,*,#1338,.F.) ;
#1833=ORIENTED_EDGE('',*,*,#1340,.T.) ;
#1834=ORIENTED_EDGE('',*,*,#1339,.F.) ;
#1835=ORIENTED_EDGE('',*,*,#1340,.F.) ;
#1836=ORIENTED_EDGE('',*,*,#1341,.T.) ;
#1837=ORIENTED_EDGE('',*,*,#1342,.T.) ;
#1838=ORIENTED_EDGE('',*,*,#1341,.F.) ;
#1839=ORIENTED_EDGE('',*,*,#1343,.F.) ;
#1840=ORIENTED_EDGE('',*,*,#1344,.T.) ;
#1841=ORIENTED_EDGE('',*,*,#1345,.T.) ;
#1842=ORIENTED_EDGE('',*,*,#1344,.F.) ;
#1843=ORIENTED_EDGE('',*,*,#1346,.T.) ;
#1844=ORIENTED_EDGE('',*,*,#1345,.F.) ;
#1845=ORIENTED_EDGE('',*,*,#1346,.F.) ;
#1846=ORIENTED_EDGE('',*,*,#1347,.T.) ;
#1847=ORIENTED_EDGE('',*,*,#1348,.T.) ;
#1848=ORIENTED_EDGE('',*,*,#1347,.F.) ;
#1849=ORIENTED_EDGE('',*,*,#1348,.F.) ;
#1850=ORIENTED_EDGE('',*,*,#1349,.T.) ;
#1851=ORIENTED_EDGE('',*,*,#1349,.F.) ;
#1852=ORIENTED_EDGE('',*,*,#1350,.T.) ;
#1853=ORIENTED_EDGE('',*,*,#1351,.T.) ;
#1854=ORIENTED_EDGE('',*,*,#1350,.F.) ;
#1855=ORIENTED_EDGE('',*,*,#1351,.F.) ;
#1856=ORIENTED_EDGE('',*,*,#1329,.T.) ;
#1857=ORIENTED_EDGE('',*,*,#1332,.T.) ;
#1858=ORIENTED_EDGE('',*,*,#1352,.T.) ;
#1859=ORIENTED_EDGE('',*,*,#1353,.T.) ;
#1860=ORIENTED_EDGE('',*,*,#1343,.T.) ;
#1861=ORIENTED_EDGE('',*,*,#1354,.T.) ;
#1862=ORIENTED_EDGE('',*,*,#1342,.F.) ;
#1863=ORIENTED_EDGE('',*,*,#1354,.F.) ;
#1864=ORIENTED_EDGE('',*,*,#1355,.F.) ;
#1865=ORIENTED_EDGE('',*,*,#1356,.F.) ;
#1866=ORIENTED_EDGE('',*,*,#1357,.F.) ;
#1867=ORIENTED_EDGE('',*,*,#1358,.F.) ;
#1868=ORIENTED_EDGE('',*,*,#1331,.F.) ;
#1869=ORIENTED_EDGE('',*,*,#1352,.F.) ;
#1870=ORIENTED_EDGE('',*,*,#1359,.T.) ;
#1871=ORIENTED_EDGE('',*,*,#1356,.T.) ;
#1872=ORIENTED_EDGE('',*,*,#1355,.T.) ;
#1873=ORIENTED_EDGE('',*,*,#1359,.F.) ;
#1874=ORIENTED_EDGE('',*,*,#1353,.F.) ;
#1875=ORIENTED_EDGE('',*,*,#1360,.T.) ;
#1876=ORIENTED_EDGE('',*,*,#1358,.T.) ;
#1877=ORIENTED_EDGE('',*,*,#1357,.T.) ;
#1878=ORIENTED_EDGE('',*,*,#1360,.F.) ;
#1879=ORIENTED_EDGE('',*,*,#1361,.F.) ;
#1880=ORIENTED_EDGE('',*,*,#1362,.T.) ;
#1881=ORIENTED_EDGE('',*,*,#1363,.T.) ;
#1882=ORIENTED_EDGE('',*,*,#1364,.F.) ;
#1883=ORIENTED_EDGE('',*,*,#1365,.T.) ;
#1884=ORIENTED_EDGE('',*,*,#1366,.T.) ;
#1885=ORIENTED_EDGE('',*,*,#1367,.T.) ;
#1886=ORIENTED_EDGE('',*,*,#1364,.T.) ;
#1887=ORIENTED_EDGE('',*,*,#1367,.F.) ;
#1888=ORIENTED_EDGE('',*,*,#1368,.T.) ;
#1889=ORIENTED_EDGE('',*,*,#1369,.T.) ;
#1890=ORIENTED_EDGE('',*,*,#1366,.F.) ;
#1891=ORIENTED_EDGE('',*,*,#1370,.F.) ;
#1892=ORIENTED_EDGE('',*,*,#1371,.T.) ;
#1893=ORIENTED_EDGE('',*,*,#1370,.T.) ;
#1894=ORIENTED_EDGE('',*,*,#1365,.F.) ;
#1895=ORIENTED_EDGE('',*,*,#1369,.F.) ;
#1896=ORIENTED_EDGE('',*,*,#1372,.T.) ;
#1897=ORIENTED_EDGE('',*,*,#1373,.T.) ;
#1898=ORIENTED_EDGE('',*,*,#1361,.T.) ;
#1899=ORIENTED_EDGE('',*,*,#1373,.F.) ;
#1900=ORIENTED_EDGE('',*,*,#1374,.T.) ;
#1901=ORIENTED_EDGE('',*,*,#1375,.T.) ;
#1902=ORIENTED_EDGE('',*,*,#1376,.T.) ;
#1903=ORIENTED_EDGE('',*,*,#1374,.F.) ;
#1904=ORIENTED_EDGE('',*,*,#1372,.F.) ;
#1905=ORIENTED_EDGE('',*,*,#1376,.F.) ;
#1906=ORIENTED_EDGE('',*,*,#1377,.T.) ;
#1907=ORIENTED_EDGE('',*,*,#1363,.F.) ;
#1908=ORIENTED_EDGE('',*,*,#1378,.T.) ;
#1909=ORIENTED_EDGE('',*,*,#1379,.T.) ;
#1910=ORIENTED_EDGE('',*,*,#1380,.T.) ;
#1911=ORIENTED_EDGE('',*,*,#1378,.F.) ;
#1912=ORIENTED_EDGE('',*,*,#1381,.F.) ;
#1913=ORIENTED_EDGE('',*,*,#1382,.F.) ;
#1914=ORIENTED_EDGE('',*,*,#1383,.T.) ;
#1915=ORIENTED_EDGE('',*,*,#1377,.F.) ;
#1916=ORIENTED_EDGE('',*,*,#1375,.F.) ;
#1917=ORIENTED_EDGE('',*,*,#1383,.F.) ;
#1918=ORIENTED_EDGE('',*,*,#1384,.T.) ;
#1919=ORIENTED_EDGE('',*,*,#1382,.T.) ;
#1920=ORIENTED_EDGE('',*,*,#1385,.F.) ;
#1921=ORIENTED_EDGE('',*,*,#1379,.F.) ;
#1922=ORIENTED_EDGE('',*,*,#1385,.T.) ;
#1923=ORIENTED_EDGE('',*,*,#1381,.T.) ;
#1924=ORIENTED_EDGE('',*,*,#1384,.F.) ;
#1925=ORIENTED_EDGE('',*,*,#1380,.F.) ;
#1926=ORIENTED_EDGE('',*,*,#1362,.F.) ;
#1927=ORIENTED_EDGE('',*,*,#1386,.T.) ;
#1928=ORIENTED_EDGE('',*,*,#1387,.T.) ;
#1929=ORIENTED_EDGE('',*,*,#1386,.F.) ;
#1930=ORIENTED_EDGE('',*,*,#1388,.F.) ;
#1931=ORIENTED_EDGE('',*,*,#1389,.T.) ;
#1932=ORIENTED_EDGE('',*,*,#1368,.F.) ;
#1933=ORIENTED_EDGE('',*,*,#1371,.F.) ;
#1934=ORIENTED_EDGE('',*,*,#1389,.F.) ;
#1935=ORIENTED_EDGE('',*,*,#1388,.T.) ;
#1936=ORIENTED_EDGE('',*,*,#1390,.T.) ;
#1937=ORIENTED_EDGE('',*,*,#1387,.F.) ;
#1938=ORIENTED_EDGE('',*,*,#1390,.F.) ;
#2096=ADVANCED_FACE('',(#550),#198,.T.) ;
#2097=ADVANCED_FACE('',(#551),#199,.T.) ;
#2098=ADVANCED_FACE('',(#552),#466,.T.) ;
#2099=ADVANCED_FACE('',(#553),#200,.T.) ;
#2100=ADVANCED_FACE('',(#554),#467,.T.) ;
#2101=ADVANCED_FACE('',(#555),#468,.F.) ;
#2102=ADVANCED_FACE('',(#556),#201,.F.) ;
#2103=ADVANCED_FACE('',(#557),#469,.F.) ;
#2104=ADVANCED_FACE('',(#558),#202,.F.) ;
#2105=ADVANCED_FACE('',(#559),#470,.F.) ;
#2106=ADVANCED_FACE('',(#560),#203,.F.) ;
#2107=ADVANCED_FACE('',(#561),#471,.F.) ;
#2108=ADVANCED_FACE('',(#562),#204,.F.) ;
#2109=ADVANCED_FACE('',(#563),#472,.F.) ;
#2110=ADVANCED_FACE('',(#564,#98),#148,.T.) ;
#2111=ADVANCED_FACE('',(#565,#99),#149,.T.) ;
#2112=ADVANCED_FACE('',(#566,#100),#150,.F.) ;
#2113=ADVANCED_FACE('',(#567,#101),#151,.F.) ;
#2114=ADVANCED_FACE('',(#568),#205,.F.) ;
#2115=ADVANCED_FACE('',(#569),#206,.T.) ;
#2116=ADVANCED_FACE('',(#570,#102),#152,.F.) ;
#2117=ADVANCED_FACE('',(#571),#473,.F.) ;
#2118=ADVANCED_FACE('',(#572),#207,.F.) ;
#2119=ADVANCED_FACE('',(#573,#103),#153,.T.) ;
#2120=ADVANCED_FACE('',(#574),#208,.T.) ;
#2121=ADVANCED_FACE('',(#575),#209,.T.) ;
#2122=ADVANCED_FACE('',(#576,#104),#154,.T.) ;
#2123=ADVANCED_FACE('',(#577),#210,.T.) ;
#2124=ADVANCED_FACE('',(#578,#105),#155,.F.) ;
#2125=ADVANCED_FACE('',(#579),#211,.T.) ;
#2126=ADVANCED_FACE('',(#580,#106,#107,#108,#109),#156,.F.) ;
#2127=ADVANCED_FACE('',(#581,#110,#111,#112),#474,.T.) ;
#2128=ADVANCED_FACE('',(#582),#212,.F.) ;
#2129=ADVANCED_FACE('',(#583),#213,.F.) ;
#2130=ADVANCED_FACE('',(#584,#113),#157,.F.) ;
#2131=ADVANCED_FACE('',(#585,#114),#158,.T.) ;
#2132=ADVANCED_FACE('',(#586),#214,.F.) ;
#2133=ADVANCED_FACE('',(#587),#55,.F.) ;
#2134=ADVANCED_FACE('',(#588),#56,.F.) ;
#2135=ADVANCED_FACE('',(#589),#215,.T.) ;
#2136=ADVANCED_FACE('',(#590),#169,.F.) ;
#2137=ADVANCED_FACE('',(#591),#216,.T.) ;
#2138=ADVANCED_FACE('',(#592),#475,.T.) ;
#2139=ADVANCED_FACE('',(#593),#57,.T.) ;
#2140=ADVANCED_FACE('',(#594),#58,.T.) ;
#2141=ADVANCED_FACE('',(#595),#217,.F.) ;
#2142=ADVANCED_FACE('',(#596),#476,.F.) ;
#2143=ADVANCED_FACE('',(#597),#170,.T.) ;
#2164=CLOSED_SHELL('',(#2096,#2097,#2098,#2099,#2100,#2101,#2102,#2103,
#2104,#2105,#2106,#2107,#2108,#2109,#2110,#2111,#2112,#2113)) ;
#2165=CLOSED_SHELL('',(#2114,#2115,#2116,#2117,#2118,#2119,#2120,#2121,
#2122,#2123,#2124,#2125,#2126,#2127,#2128,#2129)) ;
#2166=CLOSED_SHELL('',(#2130,#2131,#2132,#2133,#2134,#2135,#2136,#2137,
#2138,#2139,#2140,#2141,#2142,#2143)) ;
#2366=AXIS2_PLACEMENT_3D('',#3619,#2916,#2917) ;
#2367=AXIS2_PLACEMENT_3D('',#3620,#2918,#2919) ;
#2368=AXIS2_PLACEMENT_3D('',#3622,#2920,#2921) ;
#2369=AXIS2_PLACEMENT_3D('',#3625,#2923,#2924) ;
#2370=AXIS2_PLACEMENT_3D('',#3626,#2925,#2926) ;
#2371=AXIS2_PLACEMENT_3D('',#3628,#2927,#2928) ;
#2372=AXIS2_PLACEMENT_3D('',#3631,#2930,#2931) ;
#2373=AXIS2_PLACEMENT_3D('',#3632,#2932,#2933) ;
#2374=AXIS2_PLACEMENT_3D('',#3635,#2935,#2936) ;
#2375=AXIS2_PLACEMENT_3D('',#3636,#2937,#2938) ;
#2376=AXIS2_PLACEMENT_3D('',#3638,#2939,#2940) ;
#2377=AXIS2_PLACEMENT_3D('',#3640,#2942,#2943) ;
#2378=AXIS2_PLACEMENT_3D('',#3643,#2945,#2946) ;
#2379=AXIS2_PLACEMENT_3D('',#3644,#2947,#2948) ;
#2380=AXIS2_PLACEMENT_3D('',#3646,#2949,#2950) ;
#2381=AXIS2_PLACEMENT_3D('',#3649,#2952,#2953) ;
#2382=AXIS2_PLACEMENT_3D('',#3650,#2954,#2955) ;
#2383=AXIS2_PLACEMENT_3D('',#3652,#2956,#2957) ;
#2384=AXIS2_PLACEMENT_3D('',#3654,#2959,#2960) ;
#2385=AXIS2_PLACEMENT_3D('',#3657,#2962,#2963) ;
#2386=AXIS2_PLACEMENT_3D('',#3658,#2964,#2965) ;
#2387=AXIS2_PLACEMENT_3D('',#3660,#2966,#2967) ;
#2388=AXIS2_PLACEMENT_3D('',#3662,#2969,#2970) ;
#2389=AXIS2_PLACEMENT_3D('',#3664,#2971,#2972) ;
#2390=AXIS2_PLACEMENT_3D('',#3667,#2974,#2975) ;
#2391=AXIS2_PLACEMENT_3D('',#3668,#2976,#2977) ;
#2392=AXIS2_PLACEMENT_3D('',#3670,#2978,#2979) ;
#2393=AXIS2_PLACEMENT_3D('',#3672,#2981,#2982) ;
#2394=AXIS2_PLACEMENT_3D('',#3675,#2984,#2985) ;
#2395=AXIS2_PLACEMENT_3D('',#3676,#2986,#2987) ;
#2396=AXIS2_PLACEMENT_3D('',#3678,#2988,#2989) ;
#2397=AXIS2_PLACEMENT_3D('',#3680,#2991,#2992) ;
#2398=AXIS2_PLACEMENT_3D('',#3683,#2994,#2995) ;
#2399=AXIS2_PLACEMENT_3D('',#3684,#2996,#2997) ;
#2400=AXIS2_PLACEMENT_3D('',#3685,#2998,#2999) ;
#2401=AXIS2_PLACEMENT_3D('',#3686,#3000,#3001) ;
#2402=AXIS2_PLACEMENT_3D('',#3687,#3002,#3003) ;
#2403=AXIS2_PLACEMENT_3D('',#3688,#3004,#3005) ;
#2404=AXIS2_PLACEMENT_3D('',#3690,#3006,#3007) ;
#2405=AXIS2_PLACEMENT_3D('',#3731,#3009,#3010) ;
#2406=AXIS2_PLACEMENT_3D('',#3733,#3011,#3012) ;
#2407=AXIS2_PLACEMENT_3D('',#3736,#3014,#3015) ;
#2408=AXIS2_PLACEMENT_3D('',#3737,#3016,#3017) ;
#2409=AXIS2_PLACEMENT_3D('',#3739,#3018,#3019) ;
#2410=AXIS2_PLACEMENT_3D('',#3740,#3020,#3021) ;
#2411=AXIS2_PLACEMENT_3D('',#3742,#3022,#3023) ;
#2412=AXIS2_PLACEMENT_3D('',#3744,#3025,#3026) ;
#2413=AXIS2_PLACEMENT_3D('',#3747,#3028,#3029) ;
#2414=AXIS2_PLACEMENT_3D('',#3748,#3030,#3031) ;
#2415=AXIS2_PLACEMENT_3D('',#3750,#3032,#3033) ;
#2416=AXIS2_PLACEMENT_3D('',#3751,#3034,#3035) ;
#2417=AXIS2_PLACEMENT_3D('',#3754,#3037,#3038) ;
#2418=AXIS2_PLACEMENT_3D('',#3755,#3039,#3040) ;
#2419=AXIS2_PLACEMENT_3D('',#3757,#3041,#3042) ;
#2420=AXIS2_PLACEMENT_3D('',#3760,#3044,#3045) ;
#2421=AXIS2_PLACEMENT_3D('',#3761,#3046,#3047) ;
#2422=AXIS2_PLACEMENT_3D('',#3763,#3048,#3049) ;
#2423=AXIS2_PLACEMENT_3D('',#3764,#3050,#3051) ;
#2424=AXIS2_PLACEMENT_3D('',#3767,#3053,#3054) ;
#2425=AXIS2_PLACEMENT_3D('',#3768,#3055,#3056) ;
#2426=AXIS2_PLACEMENT_3D('',#3770,#3057,#3058) ;
#2427=AXIS2_PLACEMENT_3D('',#3771,#3059,#3060) ;
#2428=AXIS2_PLACEMENT_3D('',#3774,#3062,#3063) ;
#2429=AXIS2_PLACEMENT_3D('',#3775,#3064,#3065) ;
#2430=AXIS2_PLACEMENT_3D('',#3777,#3066,#3067) ;
#2431=AXIS2_PLACEMENT_3D('',#3779,#3068,#3069) ;
#2432=AXIS2_PLACEMENT_3D('',#3780,#3070,#3071) ;
#2433=AXIS2_PLACEMENT_3D('',#3876,#3073,#3074) ;
#2434=AXIS2_PLACEMENT_3D('',#3878,#3076,#3077) ;
#2435=AXIS2_PLACEMENT_3D('',#3880,#3079,#3080) ;
#2436=AXIS2_PLACEMENT_3D('',#3882,#3081,#3082) ;
#2437=AXIS2_PLACEMENT_3D('',#3884,#3083,#3084) ;
#2438=AXIS2_PLACEMENT_3D('',#3885,#3085,#3086) ;
#2439=AXIS2_PLACEMENT_3D('',#3887,#3087,#3088) ;
#2440=AXIS2_PLACEMENT_3D('',#3889,#3089,#3090) ;
#2441=AXIS2_PLACEMENT_3D('',#3890,#3091,#3092) ;
#2442=AXIS2_PLACEMENT_3D('',#3893,#3093,#3094) ;
#2443=AXIS2_PLACEMENT_3D('',#3894,#3095,#3096) ;
#2444=AXIS2_PLACEMENT_3D('',#4025,#3098,#3099) ;
#2445=AXIS2_PLACEMENT_3D('',#4026,#3100,#3101) ;
#2446=AXIS2_PLACEMENT_3D('',#4072,#3102,#3103) ;
#2447=AXIS2_PLACEMENT_3D('',#4073,#3104,#3105) ;
#2448=AXIS2_PLACEMENT_3D('',#4076,#3106,#3107) ;
#2449=AXIS2_PLACEMENT_3D('',#4078,#3109,#3110) ;
#2450=AXIS2_PLACEMENT_3D('',#4079,#3111,#3112) ;
#2451=AXIS2_PLACEMENT_3D('',#4082,#3113,#3114) ;
#2452=AXIS2_PLACEMENT_3D('',#4083,#3115,#3116) ;
#2453=AXIS2_PLACEMENT_3D('',#4084,#3117,#3118) ;
#2454=AXIS2_PLACEMENT_3D('',#4085,#3119,#3120) ;
#2455=AXIS2_PLACEMENT_3D('',#4089,#3122,#3123) ;
#2456=AXIS2_PLACEMENT_3D('',#4090,#3124,#3125) ;
#2457=AXIS2_PLACEMENT_3D('',#4091,#3126,#3127) ;
#2458=AXIS2_PLACEMENT_3D('',#4094,#3128,#3129) ;
#2459=AXIS2_PLACEMENT_3D('',#4095,#3130,#3131) ;
#2460=AXIS2_PLACEMENT_3D('',#4142,#3133,#3134) ;
#2461=AXIS2_PLACEMENT_3D('',#4143,#3135,#3136) ;
#2462=AXIS2_PLACEMENT_3D('',#4189,#3137,#3138) ;
#2463=AXIS2_PLACEMENT_3D('',#4192,#3140,#3141) ;
#2464=AXIS2_PLACEMENT_3D('',#4193,#3142,#3143) ;
#2465=AXIS2_PLACEMENT_3D('',#4195,#3144,#3145) ;
#2466=AXIS2_PLACEMENT_3D('',#4197,#3147,#3148) ;
#2467=AXIS2_PLACEMENT_3D('',#4198,#3149,#3150) ;
#2916=DIRECTION('axis',(0.,0.,1.)) ;
#2917=DIRECTION('refdir',(1.,0.,0.)) ;
#2918=DIRECTION('center_axis',(0.855521240266964,-0.510121382366096,0.0886542875724545)) ;
#2919=DIRECTION('ref_axis',(-0.465119843688758,-0.83240693799912,-0.301267689236459)) ;
#2920=DIRECTION('center_axis',(0.855521240266964,-0.510121382366096,0.0886542875724545)) ;
#2921=DIRECTION('ref_axis',(-0.517240562193751,-0.834304337432909,0.190783839363105)) ;
#2922=DIRECTION('',(-0.855521240266964,0.510121382366096,-0.0886542875724545)) ;
#2923=DIRECTION('center_axis',(0.855521240266964,-0.510121382366096,0.0886542875724545)) ;
#2924=DIRECTION('ref_axis',(-0.517240562193751,-0.834304337432909,0.190783839363105)) ;
#2925=DIRECTION('center_axis',(0.855521240266964,-0.510121382366096,0.0886542875724545)) ;
#2926=DIRECTION('ref_axis',(-0.465119843688758,-0.83240693799912,-0.301267689236459)) ;
#2927=DIRECTION('center_axis',(0.855521240266964,-0.510121382366096,0.0886542875724545)) ;
#2928=DIRECTION('ref_axis',(-0.517240562193751,-0.834304337432909,0.190783839363105)) ;
#2929=DIRECTION('',(-0.855521240266964,0.510121382366096,-0.0886542875724545)) ;
#2930=DIRECTION('center_axis',(0.855521240266964,-0.510121382366096,0.0886542875724545)) ;
#2931=DIRECTION('ref_axis',(-0.517240562193751,-0.834304337432909,0.190783839363105)) ;
#2932=DIRECTION('center_axis',(-0.855521240266964,0.510121382366096,-0.0886542875724545)) ;
#2933=DIRECTION('ref_axis',(-0.465119843688757,-0.83240693799912,-0.301267689236459)) ;
#2934=DIRECTION('',(0.472058877340417,-0.877268648914429,-0.0869490307936615)) ;
#2935=DIRECTION('center_axis',(-0.855521240266964,0.510121382366096,-0.0886542875724545)) ;
#2936=DIRECTION('ref_axis',(0.517240562193751,0.834304337432909,-0.190783839363105)) ;
#2937=DIRECTION('center_axis',(0.855521240266964,-0.510121382366096,0.0886542875724545)) ;
#2938=DIRECTION('ref_axis',(-0.465119843688757,-0.83240693799912,-0.301267689236459)) ;
#2939=DIRECTION('center_axis',(0.855521240266964,-0.510121382366096,0.0886542875724545)) ;
#2940=DIRECTION('ref_axis',(-0.517240562193751,-0.834304337432909,0.190783839363105)) ;
#2941=DIRECTION('',(-0.855521240266964,0.510121382366096,-0.0886542875724545)) ;
#2942=DIRECTION('center_axis',(-0.855521240266964,0.510121382366096,-0.0886542875724545)) ;
#2943=DIRECTION('ref_axis',(-0.465119843688757,-0.83240693799912,-0.301267689236459)) ;
#2944=DIRECTION('',(0.276055474905567,-0.949310879265127,-0.150340378087633)) ;
#2945=DIRECTION('center_axis',(-0.855521240266964,0.510121382366096,-0.0886542875724545)) ;
#2946=DIRECTION('ref_axis',(0.51724056219375,0.834304337432909,-0.190783839363105)) ;
#2947=DIRECTION('center_axis',(0.855521240266964,-0.510121382366096,0.0886542875724545)) ;
#2948=DIRECTION('ref_axis',(-0.465119843688758,-0.83240693799912,-0.301267689236459)) ;
#2949=DIRECTION('center_axis',(0.855521240266964,-0.510121382366096,0.0886542875724545)) ;
#2950=DIRECTION('ref_axis',(-0.517240562193751,-0.834304337432909,0.190783839363105)) ;
#2951=DIRECTION('',(0.933834265978767,0.22789030186616,0.275716473935179)) ;
#2952=DIRECTION('center_axis',(0.855521240266964,-0.510121382366096,0.0886542875724545)) ;
#2953=DIRECTION('ref_axis',(-0.517240562193751,-0.834304337432909,0.190783839363105)) ;
#2954=DIRECTION('center_axis',(0.855521240266964,-0.510121382366096,0.0886542875724545)) ;
#2955=DIRECTION('ref_axis',(-0.465119843688758,-0.83240693799912,-0.301267689236459)) ;
#2956=DIRECTION('center_axis',(0.855521240266964,-0.510121382366096,0.0886542875724545)) ;
#2957=DIRECTION('ref_axis',(-0.517240562193751,-0.834304337432909,0.190783839363105)) ;
#2958=DIRECTION('',(0.855521240266964,-0.510121382366096,0.0886542875724545)) ;
#2959=DIRECTION('center_axis',(-0.855521240266964,0.510121382366096,-0.0886542875724545)) ;
#2960=DIRECTION('ref_axis',(-0.465119843688758,-0.83240693799912,-0.301267689236459)) ;
#2961=DIRECTION('',(-0.434020190478197,0.895315978292129,0.100178706679998)) ;
#2962=DIRECTION('center_axis',(-0.855521240266964,0.510121382366096,-0.0886542875724545)) ;
#2963=DIRECTION('ref_axis',(0.517240562193751,0.834304337432909,-0.190783839363105)) ;
#2964=DIRECTION('center_axis',(0.855521240266964,-0.510121382366096,0.0886542875724545)) ;
#2965=DIRECTION('ref_axis',(-0.465119843688757,-0.83240693799912,-0.301267689236459)) ;
#2966=DIRECTION('center_axis',(0.855521240266964,-0.510121382366096,0.0886542875724545)) ;
#2967=DIRECTION('ref_axis',(-0.517240562193751,-0.834304337432909,0.190783839363105)) ;
#2968=DIRECTION('',(0.855521240266964,-0.510121382366096,0.0886542875724545)) ;
#2969=DIRECTION('center_axis',(0.855521240266964,-0.510121382366096,0.0886542875724545)) ;
#2970=DIRECTION('ref_axis',(-0.465119843688758,-0.83240693799912,-0.301267689236459)) ;
#2971=DIRECTION('center_axis',(0.855521240266964,-0.510121382366096,0.0886542875724545)) ;
#2972=DIRECTION('ref_axis',(-0.517240562193751,-0.834304337432909,0.190783839363105)) ;
#2973=DIRECTION('',(0.830566220570463,0.465824863413527,0.305232616004688)) ;
#2974=DIRECTION('center_axis',(0.855521240266964,-0.510121382366096,0.0886542875724545)) ;
#2975=DIRECTION('ref_axis',(-0.517240562193751,-0.834304337432909,0.190783839363105)) ;
#2976=DIRECTION('center_axis',(0.855521240266964,-0.510121382366096,0.0886542875724545)) ;
#2977=DIRECTION('ref_axis',(-0.465119843688758,-0.83240693799912,-0.301267689236459)) ;
#2978=DIRECTION('center_axis',(0.855521240266964,-0.510121382366096,0.0886542875724545)) ;
#2979=DIRECTION('ref_axis',(-0.517240562193751,-0.834304337432909,0.190783839363105)) ;
#2980=DIRECTION('',(0.855521240266964,-0.510121382366096,0.0886542875724545)) ;
#2981=DIRECTION('center_axis',(-0.855521240266964,0.510121382366096,-0.0886542875724545)) ;
#2982=DIRECTION('ref_axis',(-0.465119843688758,-0.83240693799912,-0.301267689236459)) ;
#2983=DIRECTION('',(-0.0249550196914587,0.975946245776617,0.216578328432755)) ;
#2984=DIRECTION('center_axis',(-0.855521240266964,0.510121382366096,-0.0886542875724545)) ;
#2985=DIRECTION('ref_axis',(0.517240562193751,0.834304337432909,-0.190783839363105)) ;
#2986=DIRECTION('center_axis',(0.855521240266964,-0.510121382366096,0.0886542875724545)) ;
#2987=DIRECTION('ref_axis',(-0.465119843688757,-0.83240693799912,-0.301267689236459)) ;
#2988=DIRECTION('center_axis',(0.855521240266964,-0.510121382366096,0.0886542875724545)) ;
#2989=DIRECTION('ref_axis',(-0.517240562193751,-0.834304337432909,0.190783839363105)) ;
#2990=DIRECTION('',(0.855521240266964,-0.510121382366096,0.0886542875724545)) ;
#2991=DIRECTION('center_axis',(-0.855521240266964,0.510121382366096,-0.0886542875724545)) ;
#2992=DIRECTION('ref_axis',(-0.465119843688757,-0.83240693799912,-0.301267689236459)) ;
#2993=DIRECTION('',(-0.276055474905567,0.949310879265127,0.150340378087633)) ;
#2994=DIRECTION('center_axis',(-0.855521240266964,0.510121382366096,-0.0886542875724545)) ;
#2995=DIRECTION('ref_axis',(0.517240562193751,0.834304337432909,-0.190783839363105)) ;
#2996=DIRECTION('center_axis',(0.855521240266964,-0.510121382366096,0.0886542875724545)) ;
#2997=DIRECTION('ref_axis',(0.0233582592152947,0.209075220419679,0.977620552122803)) ;
#2998=DIRECTION('center_axis',(0.855521240266964,-0.510121382366096,0.0886542875724545)) ;
#2999=DIRECTION('ref_axis',(0.0233582592152947,0.209075220419679,0.977620552122803)) ;
#3000=DIRECTION('center_axis',(0.855521240266964,-0.510121382366096,0.0886542875724545)) ;
#3001=DIRECTION('ref_axis',(0.0233582592152947,0.209075220419679,0.977620552122803)) ;
#3002=DIRECTION('center_axis',(0.855521240266964,-0.510121382366096,0.0886542875724545)) ;
#3003=DIRECTION('ref_axis',(0.0233582592152947,0.209075220419679,0.977620552122803)) ;
#3004=DIRECTION('center_axis',(0.855521240266964,-0.510121382366096,0.0886542875724545)) ;
#3005=DIRECTION('ref_axis',(-0.227479534154222,-0.216506038769899,0.949409393632244)) ;
#3006=DIRECTION('center_axis',(0.855521240266964,-0.510121382366096,0.0886542875724545)) ;
#3007=DIRECTION('ref_axis',(-0.517240562193751,-0.834304337432909,0.190783839363105)) ;
#3008=DIRECTION('',(0.855521240266964,-0.510121382366096,0.0886542875724545)) ;
#3009=DIRECTION('center_axis',(0.855521240266964,-0.510121382366096,0.0886542875724545)) ;
#3010=DIRECTION('ref_axis',(-0.465119843688758,-0.83240693799912,-0.301267689236459)) ;
#3011=DIRECTION('center_axis',(0.855521240266964,-0.510121382366096,0.0886542875724545)) ;
#3012=DIRECTION('ref_axis',(-0.517240562193751,-0.834304337432909,0.190783839363105)) ;
#3013=DIRECTION('',(-0.855521240266964,0.510121382366096,-0.0886542875724545)) ;
#3014=DIRECTION('center_axis',(0.855521240266964,-0.510121382366096,0.0886542875724545)) ;
#3015=DIRECTION('ref_axis',(-0.517240562193751,-0.834304337432909,0.190783839363105)) ;
#3016=DIRECTION('center_axis',(0.855521240266964,-0.510121382366096,0.0886542875724545)) ;
#3017=DIRECTION('ref_axis',(0.0233582592152947,0.209075220419679,0.977620552122803)) ;
#3018=DIRECTION('center_axis',(0.855521240266964,-0.510121382366096,0.0886542875724545)) ;
#3019=DIRECTION('ref_axis',(-0.517240562193751,-0.834304337432909,0.190783839363105)) ;
#3020=DIRECTION('center_axis',(-0.855521240266964,0.510121382366096,-0.0886542875724545)) ;
#3021=DIRECTION('ref_axis',(-0.465119843688758,-0.83240693799912,-0.301267689236459)) ;
#3022=DIRECTION('center_axis',(-0.855521240266964,0.510121382366096,-0.0886542875724545)) ;
#3023=DIRECTION('ref_axis',(0.517240562193751,0.834304337432909,-0.190783839363105)) ;
#3024=DIRECTION('',(-0.276055474905567,0.949310879265127,0.150340378087633)) ;
#3025=DIRECTION('center_axis',(0.855521240266964,-0.510121382366096,0.0886542875724545)) ;
#3026=DIRECTION('ref_axis',(-0.465119843688758,-0.83240693799912,-0.301267689236459)) ;
#3027=DIRECTION('',(0.855521240266964,-0.510121382366096,0.0886542875724545)) ;
#3028=DIRECTION('center_axis',(0.855521240266964,-0.510121382366096,0.0886542875724545)) ;
#3029=DIRECTION('ref_axis',(-0.517240562193751,-0.834304337432909,0.190783839363105)) ;
#3030=DIRECTION('center_axis',(0.855521240266964,-0.510121382366096,0.0886542875724545)) ;
#3031=DIRECTION('ref_axis',(0.0233582592152947,0.209075220419679,0.977620552122803)) ;
#3032=DIRECTION('center_axis',(0.855521240266964,-0.510121382366096,0.0886542875724545)) ;
#3033=DIRECTION('ref_axis',(-0.517240562193751,-0.834304337432909,0.190783839363105)) ;
#3034=DIRECTION('center_axis',(0.855521240266964,-0.510121382366096,0.0886542875724545)) ;
#3035=DIRECTION('ref_axis',(-0.465119843688758,-0.83240693799912,-0.301267689236459)) ;
#3036=DIRECTION('',(-0.855521240266964,0.510121382366096,-0.0886542875724545)) ;
#3037=DIRECTION('center_axis',(0.855521240266964,-0.510121382366096,0.0886542875724545)) ;
#3038=DIRECTION('ref_axis',(-0.517240562193751,-0.834304337432909,0.190783839363105)) ;
#3039=DIRECTION('center_axis',(0.855521240266964,-0.510121382366096,0.0886542875724545)) ;
#3040=DIRECTION('ref_axis',(-0.465119843688758,-0.83240693799912,-0.301267689236459)) ;
#3041=DIRECTION('center_axis',(0.855521240266964,-0.510121382366096,0.0886542875724545)) ;
#3042=DIRECTION('ref_axis',(-0.517240562193751,-0.834304337432909,0.190783839363105)) ;
#3043=DIRECTION('',(-0.855521240266964,0.510121382366096,-0.0886542875724545)) ;
#3044=DIRECTION('center_axis',(0.855521240266964,-0.510121382366096,0.0886542875724545)) ;
#3045=DIRECTION('ref_axis',(-0.517240562193751,-0.834304337432909,0.190783839363105)) ;
#3046=DIRECTION('center_axis',(0.855521240266964,-0.510121382366096,0.0886542875724545)) ;
#3047=DIRECTION('ref_axis',(0.0233582592152947,0.209075220419679,0.977620552122803)) ;
#3048=DIRECTION('center_axis',(0.855521240266964,-0.510121382366096,0.0886542875724545)) ;
#3049=DIRECTION('ref_axis',(-0.517240562193751,-0.834304337432909,0.190783839363105)) ;
#3050=DIRECTION('center_axis',(0.855521240266964,-0.510121382366096,0.0886542875724545)) ;
#3051=DIRECTION('ref_axis',(-0.465119843688757,-0.83240693799912,-0.301267689236459)) ;
#3052=DIRECTION('',(-0.855521240266964,0.510121382366096,-0.0886542875724545)) ;
#3053=DIRECTION('center_axis',(0.855521240266964,-0.510121382366096,0.0886542875724545)) ;
#3054=DIRECTION('ref_axis',(-0.517240562193751,-0.834304337432909,0.190783839363105)) ;
#3055=DIRECTION('center_axis',(0.855521240266964,-0.510121382366096,0.0886542875724545)) ;
#3056=DIRECTION('ref_axis',(0.0233582592152947,0.209075220419679,0.977620552122803)) ;
#3057=DIRECTION('center_axis',(0.855521240266964,-0.510121382366096,0.0886542875724545)) ;
#3058=DIRECTION('ref_axis',(-0.517240562193751,-0.834304337432909,0.190783839363105)) ;
#3059=DIRECTION('center_axis',(0.855521240266964,-0.510121382366096,0.0886542875724545)) ;
#3060=DIRECTION('ref_axis',(-0.465119843688758,-0.83240693799912,-0.301267689236459)) ;
#3061=DIRECTION('',(-0.855521240266964,0.510121382366096,-0.0886542875724545)) ;
#3062=DIRECTION('center_axis',(0.855521240266964,-0.510121382366096,0.0886542875724545)) ;
#3063=DIRECTION('ref_axis',(-0.517240562193751,-0.834304337432909,0.190783839363105)) ;
#3064=DIRECTION('center_axis',(0.855521240266964,-0.510121382366096,0.0886542875724545)) ;
#3065=DIRECTION('ref_axis',(0.0233582592152947,0.209075220419679,0.977620552122803)) ;
#3066=DIRECTION('center_axis',(0.855521240266964,-0.510121382366096,0.0886542875724545)) ;
#3067=DIRECTION('ref_axis',(-0.517240562193751,-0.834304337432909,0.190783839363105)) ;
#3068=DIRECTION('center_axis',(0.855521240266964,-0.510121382366096,0.0886542875724545)) ;
#3069=DIRECTION('ref_axis',(-0.517240562193751,-0.834304337432909,0.190783839363105)) ;
#3070=DIRECTION('center_axis',(-0.855521240266964,0.510121382366096,-0.0886542875724545)) ;
#3071=DIRECTION('ref_axis',(-0.465119843688758,-0.83240693799912,-0.301267689236459)) ;
#3072=DIRECTION('',(0.220742469906792,-0.961054902255409,-0.166271575533209)) ;
#3073=DIRECTION('center_axis',(0.855521240266964,-0.510121382366096,0.0886542875724545)) ;
#3074=DIRECTION('ref_axis',(-0.289065833361634,-0.612632535208754,-0.735610169034278)) ;
#3075=DIRECTION('',(0.855521240266964,-0.510121382366096,0.0886542875724545)) ;
#3076=DIRECTION('center_axis',(0.855521240266964,-0.510121382366096,0.0886542875724545)) ;
#3077=DIRECTION('ref_axis',(0.516545367515822,0.829138573978605,-0.213799224597913)) ;
#3078=DIRECTION('',(0.855521240266964,-0.510121382366096,0.0886542875724545)) ;
#3079=DIRECTION('center_axis',(0.855521240266964,-0.510121382366096,0.0886542875724545)) ;
#3080=DIRECTION('ref_axis',(0.0233582592152947,0.209075220419679,0.977620552122803)) ;
#3081=DIRECTION('center_axis',(0.855521240266964,-0.510121382366096,0.0886542875724545)) ;
#3082=DIRECTION('ref_axis',(-0.517240562193751,-0.834304337432909,0.190783839363105)) ;
#3083=DIRECTION('center_axis',(0.855521240266964,-0.510121382366096,0.0886542875724545)) ;
#3084=DIRECTION('ref_axis',(-0.517240562193751,-0.834304337432909,0.190783839363105)) ;
#3085=DIRECTION('center_axis',(0.855521240266964,-0.510121382366096,0.0886542875724545)) ;
#3086=DIRECTION('ref_axis',(0.0233582592152947,0.209075220419679,0.977620552122803)) ;
#3087=DIRECTION('center_axis',(0.855521240266964,-0.510121382366096,0.0886542875724545)) ;
#3088=DIRECTION('ref_axis',(-0.517240562193751,-0.834304337432909,0.190783839363105)) ;
#3089=DIRECTION('center_axis',(0.855521240266964,-0.510121382366096,0.0886542875724545)) ;
#3090=DIRECTION('ref_axis',(-0.517240562193751,-0.834304337432909,0.190783839363105)) ;
#3091=DIRECTION('center_axis',(0.855521240266964,-0.510121382366096,0.0886542875724545)) ;
#3092=DIRECTION('ref_axis',(-0.465119843688758,-0.83240693799912,-0.301267689236459)) ;
#3093=DIRECTION('center_axis',(0.855521240266964,-0.510121382366096,0.0886542875724545)) ;
#3094=DIRECTION('ref_axis',(-0.517240562193751,-0.834304337432909,0.190783839363105)) ;
#3095=DIRECTION('center_axis',(0.855521240266964,-0.510121382366096,0.0886542875724545)) ;
#3096=DIRECTION('ref_axis',(-0.517240562193751,-0.834304337432909,0.190783839363105)) ;
#3097=DIRECTION('',(0.855521240266964,-0.510121382366096,0.0886542875724545)) ;
#3098=DIRECTION('center_axis',(-0.22747999965104,-0.216506928060168,0.949409079301811)) ;
#3099=DIRECTION('ref_axis',(0.421816601389418,0.856842394307428,0.296465623824745)) ;
#3100=DIRECTION('center_axis',(0.227479534082472,0.216506038642441,-0.949409393678501)) ;
#3101=DIRECTION('ref_axis',(-0.507262223798798,-0.805894130045609,-0.305318992964293)) ;
#3102=DIRECTION('center_axis',(-0.855521239991043,0.510121383082549,-0.088654286112606)) ;
#3103=DIRECTION('ref_axis',(-0.46511984467153,-0.832406937392223,-0.301267689396044)) ;
#3104=DIRECTION('center_axis',(0.855521240266964,-0.510121382366096,0.0886542875724545)) ;
#3105=DIRECTION('ref_axis',(-0.465119843688758,-0.83240693799912,-0.301267689236459)) ;
#3106=DIRECTION('center_axis',(0.855521240266964,-0.510121382366096,0.0886542875724545)) ;
#3107=DIRECTION('ref_axis',(-0.517240562193751,-0.834304337432909,0.190783839363105)) ;
#3108=DIRECTION('',(-0.855521240266964,0.510121382366096,-0.0886542875724545)) ;
#3109=DIRECTION('center_axis',(0.855521240266964,-0.510121382366096,0.0886542875724545)) ;
#3110=DIRECTION('ref_axis',(-0.517240562193751,-0.834304337432909,0.190783839363105)) ;
#3111=DIRECTION('center_axis',(0.855521240266964,-0.510121382366096,0.0886542875724545)) ;
#3112=DIRECTION('ref_axis',(0.509998973339437,0.80069041569811,-0.314318159516608)) ;
#3113=DIRECTION('center_axis',(0.855521240266964,-0.510121382366096,0.0886542875724545)) ;
#3114=DIRECTION('ref_axis',(-0.517240562193751,-0.834304337432909,0.190783839363105)) ;
#3115=DIRECTION('center_axis',(0.0893557756655708,0.314119457312169,0.945169038793121)) ;
#3116=DIRECTION('ref_axis',(-0.509998973339439,-0.800690415698109,0.314318159516608)) ;
#3117=DIRECTION('center_axis',(0.855521240266964,-0.510121382366096,0.0886542875724545)) ;
#3118=DIRECTION('ref_axis',(-0.517240562193751,-0.834304337432909,0.190783839363105)) ;
#3119=DIRECTION('center_axis',(0.855521240266964,-0.510121382366096,0.0886542875724545)) ;
#3120=DIRECTION('ref_axis',(-0.465119843688757,-0.832406937999119,-0.301267689236459)) ;
#3121=DIRECTION('',(-0.855521240266964,0.510121382366096,-0.0886542875724545)) ;
#3122=DIRECTION('center_axis',(0.855521240266964,-0.510121382366096,0.0886542875724545)) ;
#3123=DIRECTION('ref_axis',(-0.517240562193751,-0.834304337432909,0.190783839363105)) ;
#3124=DIRECTION('center_axis',(0.855521240266964,-0.510121382366096,0.0886542875724545)) ;
#3125=DIRECTION('ref_axis',(-0.517240562193751,-0.834304337432909,0.190783839363105)) ;
#3126=DIRECTION('center_axis',(0.855521240266964,-0.510121382366096,0.0886542875724545)) ;
#3127=DIRECTION('ref_axis',(-0.465119843688758,-0.83240693799912,-0.301267689236459)) ;
#3128=DIRECTION('center_axis',(0.855521240266964,-0.510121382366096,0.0886542875724545)) ;
#3129=DIRECTION('ref_axis',(-0.517240562193751,-0.834304337432909,0.190783839363105)) ;
#3130=DIRECTION('center_axis',(0.855521240266964,-0.510121382366096,0.0886542875724545)) ;
#3131=DIRECTION('ref_axis',(-0.517240562193751,-0.834304337432909,0.190783839363105)) ;
#3132=DIRECTION('',(-0.877680816263419,0.467916504938536,-0.103588267527187)) ;
#3133=DIRECTION('center_axis',(0.227477963935797,0.216503188953687,-0.94941041973243)) ;
#3134=DIRECTION('ref_axis',(0.465119508114888,0.832408339490032,0.301264334959204)) ;
#3135=DIRECTION('center_axis',(-0.227479533901985,-0.216506038339706,0.949409393790783)) ;
#3136=DIRECTION('ref_axis',(-0.465119843754982,-0.832406938143867,-0.301267688734278)) ;
#3137=DIRECTION('center_axis',(0.855521240266964,-0.510121382366096,0.0886542875724545)) ;
#3138=DIRECTION('ref_axis',(-0.465119843688758,-0.83240693799912,-0.301267689236459)) ;
#3139=DIRECTION('',(0.855521240266964,-0.510121382366096,0.0886542875724545)) ;
#3140=DIRECTION('center_axis',(0.855521240266964,-0.510121382366096,0.0886542875724545)) ;
#3141=DIRECTION('ref_axis',(-0.517240562193751,-0.834304337432909,0.190783839363105)) ;
#3142=DIRECTION('center_axis',(0.855521240266964,-0.510121382366096,0.0886542875724545)) ;
#3143=DIRECTION('ref_axis',(-0.465119843688758,-0.83240693799912,-0.301267689236459)) ;
#3144=DIRECTION('center_axis',(0.855521240266964,-0.510121382366096,0.0886542875724545)) ;
#3145=DIRECTION('ref_axis',(-0.517240562193751,-0.834304337432909,0.190783839363105)) ;
#3146=DIRECTION('',(0.877680816263419,-0.467916504938536,0.103588267527187)) ;
#3147=DIRECTION('center_axis',(-0.855521240266964,0.510121382366096,-0.0886542875724545)) ;
#3148=DIRECTION('ref_axis',(-0.465119843688759,-0.83240693799912,-0.301267689236457)) ;
#3149=DIRECTION('center_axis',(0.227479534154222,0.216506038769899,-0.949409393632244)) ;
#3150=DIRECTION('ref_axis',(0.465119843688757,0.83240693799912,0.301267689236458)) ;
#3619=CARTESIAN_POINT('',(0.,0.,0.)) ;
#3620=CARTESIAN_POINT('Origin',(-408.672905494227,141.363671355823,-57.1369266933493)) ;
#3621=CARTESIAN_POINT('',(-408.181726471869,148.672541235612,-55.3525040279398)) ;
#3622=CARTESIAN_POINT('Origin',(-411.367797401137,142.970553710317,-57.4161876992097)) ;
#3623=CARTESIAN_POINT('',(-420.672336579767,156.120313418157,-56.6468566264977)) ;
#3624=CARTESIAN_POINT('',(-405.486834564959,147.065658881117,-55.0732430220794)) ;
#3625=CARTESIAN_POINT('Origin',(-423.858407509036,150.418325892863,-58.7105402977676)) ;
#3626=CARTESIAN_POINT('Origin',(-408.672905494227,141.363671355823,-57.1369266933493)) ;
#3627=CARTESIAN_POINT('',(-405.668306122096,146.230582638267,-55.3071569860444)) ;
#3628=CARTESIAN_POINT('Origin',(-408.459025184229,141.236141010272,-57.1147631214633)) ;
#3629=CARTESIAN_POINT('',(-408.577078339004,147.964995338312,-55.6085815637908)) ;
#3630=CARTESIAN_POINT('',(-405.882186432094,146.358112983818,-55.3293205579304)) ;
#3631=CARTESIAN_POINT('Origin',(-411.367797401137,142.970553710317,-57.4161876992097)) ;
#3632=CARTESIAN_POINT('Origin',(-403.75365836276,138.430473407259,-56.6271645398148)) ;
#3633=CARTESIAN_POINT('',(-402.590858753538,140.511490752257,-55.8739953167236)) ;
#3634=CARTESIAN_POINT('',(-402.590858753538,140.511490752257,-55.8739953167236)) ;
#3635=CARTESIAN_POINT('Origin',(-403.75365836276,138.430473407259,-56.6271645398148)) ;
#3636=CARTESIAN_POINT('Origin',(-408.672905494227,141.363671355823,-57.1369266933493)) ;
#3637=CARTESIAN_POINT('',(-392.581260242414,134.543070578573,-54.8367401521258)) ;
#3638=CARTESIAN_POINT('Origin',(-393.744059851636,132.462053233575,-55.589909375217)) ;
#3639=CARTESIAN_POINT('',(-407.510105885005,143.444688700821,-56.3837574702581)) ;
#3640=CARTESIAN_POINT('Origin',(-393.487403479556,132.309016818865,-55.5633130889452)) ;
#3641=CARTESIAN_POINT('',(-392.464139823441,134.140312082463,-54.900524172625)) ;
#3642=CARTESIAN_POINT('',(-392.464139823441,134.140312082463,-54.9005241726249)) ;
#3643=CARTESIAN_POINT('Origin',(-393.487403479556,132.309016818865,-55.5633130889452)) ;
#3644=CARTESIAN_POINT('Origin',(-393.744059851636,132.462053233575,-55.589909375217)) ;
#3645=CARTESIAN_POINT('',(-393.278940007947,133.294460171574,-55.2886416859805)) ;
#3646=CARTESIAN_POINT('Origin',(-393.744059851636,132.462053233575,-55.589909375217)) ;
#3647=CARTESIAN_POINT('',(-392.882747682761,133.391145838264,-55.1716650929378)) ;
#3648=CARTESIAN_POINT('',(-393.278940007947,133.294460171574,-55.2886416859805)) ;
#3649=CARTESIAN_POINT('Origin',(-393.487403479556,132.309016818865,-55.5633130889452)) ;
#3650=CARTESIAN_POINT('Origin',(-408.672905494227,141.363671355823,-57.1369266933493)) ;
#3651=CARTESIAN_POINT('',(-404.999580999606,140.28312310999,-56.5032054257232)) ;
#3652=CARTESIAN_POINT('Origin',(-405.464700843295,139.450716171991,-56.8044731149597)) ;
#3653=CARTESIAN_POINT('',(-408.207785650538,142.196078293822,-56.8356590041128)) ;
#3654=CARTESIAN_POINT('Origin',(-405.464700843295,139.450716171991,-56.8044731149597)) ;
#3655=CARTESIAN_POINT('',(-407.458827108158,145.35616437361,-55.9355726289835)) ;
#3656=CARTESIAN_POINT('',(-404.999580999606,140.28312310999,-56.5032054257232)) ;
#3657=CARTESIAN_POINT('Origin',(-409.435586443835,141.818434887114,-57.2159603082382)) ;
#3658=CARTESIAN_POINT('Origin',(-408.672905494227,141.363671355823,-57.1369266933493)) ;
#3659=CARTESIAN_POINT('',(-408.193308329086,145.794113261501,-56.0116840173532)) ;
#3660=CARTESIAN_POINT('Origin',(-410.170067664763,142.256383775005,-57.2920716966082)) ;
#3661=CARTESIAN_POINT('',(-406.69614615855,144.90140084232,-55.8565390140943)) ;
#3662=CARTESIAN_POINT('Origin',(-410.457044142834,142.427499149831,-57.3218099357261)) ;
#3663=CARTESIAN_POINT('',(-408.464935852315,145.992698065281,-56.0314804227262)) ;
#3664=CARTESIAN_POINT('Origin',(-410.457044142834,142.427499149831,-57.3218099357261)) ;
#3665=CARTESIAN_POINT('',(-407.907724745062,146.305211121435,-55.8267056561618)) ;
#3666=CARTESIAN_POINT('',(-408.464935852315,145.992698065282,-56.0314804227263)) ;
#3667=CARTESIAN_POINT('Origin',(-410.170067664763,142.256383775005,-57.2920716966082)) ;
#3668=CARTESIAN_POINT('Origin',(-408.672905494227,141.363671355823,-57.1369266933493)) ;
#3669=CARTESIAN_POINT('',(-419.801105043013,152.752112123184,-57.2062028680609)) ;
#3670=CARTESIAN_POINT('Origin',(-421.793213333533,149.186913207734,-58.4965323810607)) ;
#3671=CARTESIAN_POINT('',(-406.680797203708,144.928870271273,-55.8465971803495)) ;
#3672=CARTESIAN_POINT('Origin',(-421.793213333533,149.186913207734,-58.4965323810607)) ;
#3673=CARTESIAN_POINT('',(-419.821765810054,153.560117818126,-57.0268932764394)) ;
#3674=CARTESIAN_POINT('',(-419.801105043014,152.752112123185,-57.2062028680609)) ;
#3675=CARTESIAN_POINT('Origin',(-422.147365028502,149.39808312813,-58.5332317226227)) ;
#3676=CARTESIAN_POINT('Origin',(-408.672905494227,141.363671355823,-57.1369266933493)) ;
#3677=CARTESIAN_POINT('',(-421.361704042538,154.478336306385,-57.1864709940707)) ;
#3678=CARTESIAN_POINT('Origin',(-423.687303260982,150.31630161639,-58.6928094402531)) ;
#3679=CARTESIAN_POINT('',(-406.347306275783,145.525706045819,-55.6305882471669)) ;
#3680=CARTESIAN_POINT('Origin',(-423.687303260982,150.31630161639,-58.6928094402531)) ;
#3681=CARTESIAN_POINT('',(-421.439784321854,154.746841970458,-57.1439483137379)) ;
#3682=CARTESIAN_POINT('',(-421.361704042538,154.478336306386,-57.1864709940707)) ;
#3683=CARTESIAN_POINT('Origin',(-423.858407509036,150.418325892863,-58.7105402977676)) ;
#3684=CARTESIAN_POINT('Origin',(-414.910895252164,137.255568998901,-56.1093183995723)) ;
#3685=CARTESIAN_POINT('Origin',(-394.625332716382,130.473547276512,-55.1435886423464)) ;
#3686=CARTESIAN_POINT('Origin',(-412.368340054087,138.710590340914,-56.481240379315)) ;
#3687=CARTESIAN_POINT('Origin',(-426.548058432443,146.079943338211,-57.7184643330794)) ;
#3688=CARTESIAN_POINT('Origin',(-419.401620616319,145.13262479315,-57.6866191692542)) ;
#3689=CARTESIAN_POINT('',(-419.418928880099,145.248588743018,-57.9803074161011)) ;
#3690=CARTESIAN_POINT('Origin',(-419.487172740346,145.183636931387,-57.6954845980114)) ;
#3691=CARTESIAN_POINT('',(-412.553607560257,141.155005746794,-57.2688812797066)) ;
#3692=CARTESIAN_POINT('',(-419.333376756073,145.197576604781,-57.9714419873439)) ;
#3693=CARTESIAN_POINT('Ctrl Pts',(-412.676919232686,141.2339336726,-56.7092671151722)) ;
#3694=CARTESIAN_POINT('Ctrl Pts',(-412.726221526063,141.220486185843,-56.7000347274095)) ;
#3695=CARTESIAN_POINT('Ctrl Pts',(-412.780237048048,141.203418744776,-56.6975093825531)) ;
#3696=CARTESIAN_POINT('Ctrl Pts',(-412.883694241173,141.165398454256,-56.7113289821998)) ;
#3697=CARTESIAN_POINT('Ctrl Pts',(-412.933141915367,141.144467080632,-56.7276880576375)) ;
#3698=CARTESIAN_POINT('Ctrl Pts',(-413.009081951286,141.107464069561,-56.7731191552882)) ;
#3699=CARTESIAN_POINT('Ctrl Pts',(-413.041997367993,141.089077365977,-56.8026459175359)) ;
#3700=CARTESIAN_POINT('Ctrl Pts',(-413.076606466844,141.064863662361,-56.8567831525088)) ;
#3701=CARTESIAN_POINT('Ctrl Pts',(-413.085785778931,141.057328086883,-56.8764350833939)) ;
#3702=CARTESIAN_POINT('Ctrl Pts',(-413.098405249366,141.044070922671,-56.9175614950294)) ;
#3703=CARTESIAN_POINT('Ctrl Pts',(-413.101846592404,141.038349309035,-56.9390356042263)) ;
#3704=CARTESIAN_POINT('Ctrl Pts',(-413.102874041078,141.029152816437,-56.9820377359598)) ;
#3705=CARTESIAN_POINT('Ctrl Pts',(-413.100473082469,141.025562152055,-57.0041071627164)) ;
#3706=CARTESIAN_POINT('Ctrl Pts',(-413.089875154383,141.020724885159,-57.0475889973176)) ;
#3707=CARTESIAN_POINT('Ctrl Pts',(-413.081676984783,141.019478445686,-57.0690011307828)) ;
#3708=CARTESIAN_POINT('Ctrl Pts',(-413.04981465685,141.019106338779,-57.1298253609199)) ;
#3709=CARTESIAN_POINT('Ctrl Pts',(-413.018463263424,141.02349377516,-57.1657581557835)) ;
#3710=CARTESIAN_POINT('Ctrl Pts',(-412.945042397752,141.037948184903,-57.2257626809506)) ;
#3711=CARTESIAN_POINT('Ctrl Pts',(-412.896600259782,141.049879199996,-57.251488628588)) ;
#3712=CARTESIAN_POINT('Ctrl Pts',(-412.794258470493,141.077915728419,-57.2843523756985)) ;
#3713=CARTESIAN_POINT('Ctrl Pts',(-412.740353258286,141.09399580819,-57.2914945502996)) ;
#3714=CARTESIAN_POINT('Ctrl Pts',(-412.645590273407,141.123769060528,-57.2902200682869)) ;
#3715=CARTESIAN_POINT('Ctrl Pts',(-412.596828621117,141.139796832197,-57.2830215450146)) ;
#3716=CARTESIAN_POINT('Ctrl Pts',(-412.505050414036,141.172088889752,-57.2530168351479)) ;
#3717=CARTESIAN_POINT('Ctrl Pts',(-412.462009546431,141.188351512697,-57.2302832756091)) ;
#3718=CARTESIAN_POINT('Ctrl Pts',(-412.402535340985,141.213954732135,-57.1811079957144)) ;
#3719=CARTESIAN_POINT('Ctrl Pts',(-412.378983312568,141.225294776528,-57.1548298739571)) ;
#3720=CARTESIAN_POINT('Ctrl Pts',(-412.345902244053,141.245901273597,-57.094749541473)) ;
#3721=CARTESIAN_POINT('Ctrl Pts',(-412.336529826198,141.255181308432,-57.0608658812438)) ;
#3722=CARTESIAN_POINT('Ctrl Pts',(-412.334946143032,141.269356547435,-56.9945834927675)) ;
#3723=CARTESIAN_POINT('Ctrl Pts',(-412.342670191364,141.274830746562,-56.9594774261293)) ;
#3724=CARTESIAN_POINT('Ctrl Pts',(-412.372769961544,141.280909269161,-56.8947805439396)) ;
#3725=CARTESIAN_POINT('Ctrl Pts',(-412.394985379514,141.281532964064,-56.8651170892932)) ;
#3726=CARTESIAN_POINT('Ctrl Pts',(-412.451898726647,141.278851487698,-56.8071119626716)) ;
#3727=CARTESIAN_POINT('Ctrl Pts',(-412.493695520927,141.273724322324,-56.7777769310266)) ;
#3728=CARTESIAN_POINT('Ctrl Pts',(-412.583687827021,141.257417516029,-56.7330357665052)) ;
#3729=CARTESIAN_POINT('Ctrl Pts',(-412.631910958312,141.246209940744,-56.7176954014261)) ;
#3730=CARTESIAN_POINT('Ctrl Pts',(-412.676919232686,141.2339336726,-56.7092671151722)) ;
#3731=CARTESIAN_POINT('Origin',(-414.148241431988,144.628448202997,-57.7043141338184)) ;
#3732=CARTESIAN_POINT('',(-417.692863650504,148.184665926882,-57.7426394325392)) ;
#3733=CARTESIAN_POINT('Origin',(-418.2975194473,147.102536907483,-58.1342874285466)) ;
#3734=CARTESIAN_POINT('',(-420.259427371306,149.71503007398,-58.0086022952566)) ;
#3735=CARTESIAN_POINT('',(-413.543585635193,145.710577222396,-57.312666137811)) ;
#3736=CARTESIAN_POINT('Origin',(-420.864083168101,148.632901054581,-58.400250291264)) ;
#3737=CARTESIAN_POINT('Origin',(-421.536495898953,147.548305415918,-58.1522313000919)) ;
#3738=CARTESIAN_POINT('',(-420.538499277519,149.215585911181,-58.1893629087985)) ;
#3739=CARTESIAN_POINT('Origin',(-420.864083168101,148.632901054581,-58.400250291264)) ;
#3740=CARTESIAN_POINT('Origin',(-420.521874671994,148.428852501635,-58.364788576235)) ;
#3741=CARTESIAN_POINT('',(-420.382338718888,148.678574583035,-58.2744082694641)) ;
#3742=CARTESIAN_POINT('Origin',(-420.521874671994,148.428852501635,-58.364788576235)) ;
#3743=CARTESIAN_POINT('',(-420.382338718887,148.678574583035,-58.2744082694641)) ;
#3744=CARTESIAN_POINT('Origin',(-414.148241431988,144.628448202997,-57.7043141338184)) ;
#3745=CARTESIAN_POINT('',(-407.292863742802,140.873717432833,-56.9179976696054)) ;
#3746=CARTESIAN_POINT('',(-414.008705478881,144.878170284397,-57.6139338270475)) ;
#3747=CARTESIAN_POINT('Origin',(-407.432399695909,140.623995351433,-57.0083779763764)) ;
#3748=CARTESIAN_POINT('Origin',(-407.872054173773,139.914836664615,-56.8462117129177)) ;
#3749=CARTESIAN_POINT('',(-407.037047828773,141.331541248732,-56.752300440525)) ;
#3750=CARTESIAN_POINT('Origin',(-407.432399695909,140.623995351433,-57.0083779763764)) ;
#3751=CARTESIAN_POINT('Origin',(-414.148241431988,144.628448202997,-57.7043141338184)) ;
#3752=CARTESIAN_POINT('',(-410.031372169708,143.116966087014,-57.0625904470286)) ;
#3753=CARTESIAN_POINT('',(-413.752889564853,145.335994100296,-57.4482365979674)) ;
#3754=CARTESIAN_POINT('Origin',(-410.426724036843,142.409420189714,-57.31866798288)) ;
#3755=CARTESIAN_POINT('Origin',(-414.148241431988,144.628448202997,-57.7043141338184)) ;
#3756=CARTESIAN_POINT('',(-410.828799568389,146.58875613729,-56.4619379762644)) ;
#3757=CARTESIAN_POINT('Origin',(-412.479975013484,143.633711507393,-57.5314382730539)) ;
#3758=CARTESIAN_POINT('',(-412.197633552816,147.404950349076,-56.6037848363803)) ;
#3759=CARTESIAN_POINT('',(-412.497065986893,147.583492832894,-56.6348138370289)) ;
#3760=CARTESIAN_POINT('Origin',(-413.848808997911,144.449905719179,-57.6732851331698)) ;
#3761=CARTESIAN_POINT('Origin',(-416.047081387235,140.904112285089,-56.8624538158766)) ;
#3762=CARTESIAN_POINT('',(-411.872049662236,147.987635205673,-56.3928974539119)) ;
#3763=CARTESIAN_POINT('Origin',(-413.848808997911,144.449905719179,-57.6732851331698)) ;
#3764=CARTESIAN_POINT('Origin',(-414.148241431988,144.628448202997,-57.7043141338184)) ;
#3765=CARTESIAN_POINT('',(-413.754196390824,149.109902246878,-56.5879368865713)) ;
#3766=CARTESIAN_POINT('',(-412.171482096311,148.166177689494,-56.4239264545634)) ;
#3767=CARTESIAN_POINT('Origin',(-415.730955726499,145.572172760384,-57.8683245658292)) ;
#3768=CARTESIAN_POINT('Origin',(-417.28267741308,143.069259748086,-57.2959730477399)) ;
#3769=CARTESIAN_POINT('',(-414.335596195432,148.069393574382,-56.9645214981198)) ;
#3770=CARTESIAN_POINT('Origin',(-415.730955726499,145.572172760384,-57.8683245658292)) ;
#3771=CARTESIAN_POINT('Origin',(-414.148241431988,144.628448202997,-57.7043141338184)) ;
#3772=CARTESIAN_POINT('',(-416.902159916234,149.59975772148,-57.2304843608372)) ;
#3773=CARTESIAN_POINT('',(-412.752881900922,147.125669016995,-56.800511066109)) ;
#3774=CARTESIAN_POINT('Origin',(-418.2975194473,147.102536907483,-58.1342874285466)) ;
#3775=CARTESIAN_POINT('Origin',(-419.849241133881,144.599623895184,-57.5619359104573)) ;
#3776=CARTESIAN_POINT('',(-417.662499396266,147.829328416068,-60.0802875299202)) ;
#3777=CARTESIAN_POINT('Origin',(-417.749219146275,147.645538655506,-60.3009705806305)) ;
#3778=CARTESIAN_POINT('',(-417.811130065534,148.229693563362,-56.3422673396185)) ;
#3779=CARTESIAN_POINT('Origin',(-417.656166455279,148.478435135556,-56.4064071069979)) ;
#3780=CARTESIAN_POINT('Origin',(-410.426724036843,142.409420189714,-57.31866798288)) ;
#3781=CARTESIAN_POINT('',(-410.031372169707,143.116966087013,-57.062590447029)) ;
#3782=CARTESIAN_POINT('',(-411.18794426283,143.497751214042,-59.8327482012076)) ;
#3783=CARTESIAN_POINT('',(-410.797178076421,143.735745419843,-59.3688613935254)) ;
#3784=CARTESIAN_POINT('Ctrl Pts',(-411.187944262825,143.497751214042,-59.8327482012091)) ;
#3785=CARTESIAN_POINT('Ctrl Pts',(-411.192211586621,143.519120254733,-59.8488679240781)) ;
#3786=CARTESIAN_POINT('Ctrl Pts',(-411.194834914286,143.541552441395,-59.8632297300923)) ;
#3787=CARTESIAN_POINT('Ctrl Pts',(-411.197337245685,143.603213566409,-59.8959336495249)) ;
#3788=CARTESIAN_POINT('Ctrl Pts',(-411.193883331881,143.64812965929,-59.9121798889122)) ;
#3789=CARTESIAN_POINT('Ctrl Pts',(-411.179107650862,143.714566933321,-59.9212739114798)) ;
#3790=CARTESIAN_POINT('Ctrl Pts',(-411.172638140343,143.736590905115,-59.9218511079237)) ;
#3791=CARTESIAN_POINT('Ctrl Pts',(-411.156996770963,143.778597502592,-59.917706412113)) ;
#3792=CARTESIAN_POINT('Ctrl Pts',(-411.147825724058,143.798580515091,-59.9129853761654)) ;
#3793=CARTESIAN_POINT('Ctrl Pts',(-411.127608522821,143.834960290994,-59.898751924725)) ;
#3794=CARTESIAN_POINT('Ctrl Pts',(-411.116307830456,143.851815082021,-59.8890603076353)) ;
#3795=CARTESIAN_POINT('Ctrl Pts',(-411.092171126716,143.881387006667,-59.8652001740172)) ;
#3796=CARTESIAN_POINT('Ctrl Pts',(-411.079334607066,143.894103207011,-59.8510310149819)) ;
#3797=CARTESIAN_POINT('Ctrl Pts',(-411.040061826278,143.924923258829,-59.8038854269408)) ;
#3798=CARTESIAN_POINT('Ctrl Pts',(-411.012740311386,143.935385909337,-59.7659724610472)) ;
#3799=CARTESIAN_POINT('Ctrl Pts',(-410.959733804494,143.939902382881,-59.6861601298485)) ;
#3800=CARTESIAN_POINT('Ctrl Pts',(-410.931059528474,143.931407156765,-59.638658221865)) ;
#3801=CARTESIAN_POINT('Ctrl Pts',(-410.879598412631,143.89577229749,-59.5468877200924)) ;
#3802=CARTESIAN_POINT('Ctrl Pts',(-410.856788210741,143.868635778449,-59.5026310194625)) ;
#3803=CARTESIAN_POINT('Ctrl Pts',(-410.822644525485,143.810126455096,-59.4312342708784)) ;
#3804=CARTESIAN_POINT('Ctrl Pts',(-410.807844544746,143.775206429643,-59.3975338994376)) ;
#3805=CARTESIAN_POINT('Ctrl Pts',(-410.797178076421,143.735745419843,-59.3688613935255)) ;
#3806=CARTESIAN_POINT('Ctrl Pts',(-410.797178076421,143.735745419843,-59.3688613935255)) ;
#3807=CARTESIAN_POINT('Ctrl Pts',(-410.796967543334,143.73496654459,-59.3682954600788)) ;
#3808=CARTESIAN_POINT('Ctrl Pts',(-410.796758323441,143.734186086876,-59.3677313390647)) ;
#3809=CARTESIAN_POINT('Ctrl Pts',(-410.785845388505,143.692982926168,-59.3381327400731)) ;
#3810=CARTESIAN_POINT('Ctrl Pts',(-410.779463747391,143.647942683771,-59.3143744754051)) ;
#3811=CARTESIAN_POINT('Ctrl Pts',(-410.778761937223,143.570997592292,-59.2881090138335)) ;
#3812=CARTESIAN_POINT('Ctrl Pts',(-410.781594428872,143.534892229704,-59.2802214213014)) ;
#3813=CARTESIAN_POINT('Ctrl Pts',(-410.796594740226,143.464927094214,-59.277305663745)) ;
#3814=CARTESIAN_POINT('Ctrl Pts',(-410.808892850738,143.431090464959,-59.2823951324787)) ;
#3815=CARTESIAN_POINT('Ctrl Pts',(-410.840055128798,143.375015606763,-59.3043342113034)) ;
#3816=CARTESIAN_POINT('Ctrl Pts',(-410.860192135688,143.350486971278,-59.3220799344001)) ;
#3817=CARTESIAN_POINT('Ctrl Pts',(-410.903855103505,143.314890663075,-59.3662962125199)) ;
#3818=CARTESIAN_POINT('Ctrl Pts',(-410.927323217479,143.303669487857,-59.3927001361998)) ;
#3819=CARTESIAN_POINT('Ctrl Pts',(-410.978415270172,143.289940024074,-59.4544416788403)) ;
#3820=CARTESIAN_POINT('Ctrl Pts',(-411.009276655513,143.29093027168,-59.4954343394395)) ;
#3821=CARTESIAN_POINT('Ctrl Pts',(-411.065829426459,143.308536877846,-59.5782479277446)) ;
#3822=CARTESIAN_POINT('Ctrl Pts',(-411.091495321212,143.32522544883,-59.6200708925011)) ;
#3823=CARTESIAN_POINT('Ctrl Pts',(-411.1121902565,143.345763576877,-59.6574526056856)) ;
#3824=CARTESIAN_POINT('Ctrl Pts',(-411.134859594198,143.368261147123,-59.6984007250256)) ;
#3825=CARTESIAN_POINT('Ctrl Pts',(-411.155499220532,143.399303501171,-59.7411292822976)) ;
#3826=CARTESIAN_POINT('Ctrl Pts',(-411.177665344724,143.455729666604,-59.7984489428495)) ;
#3827=CARTESIAN_POINT('Ctrl Pts',(-411.183640679057,143.476200597996,-59.816491507082)) ;
#3828=CARTESIAN_POINT('Ctrl Pts',(-411.187944262825,143.497751214042,-59.8327482012091)) ;
#3829=CARTESIAN_POINT('',(-410.853208211569,144.763179026854,-55.7816414442377)) ;
#3830=CARTESIAN_POINT('',(-410.945808745689,144.136110567136,-55.6308412032236)) ;
#3831=CARTESIAN_POINT('Ctrl Pts',(-410.853208211571,144.76317902685,-55.7816414442362)) ;
#3832=CARTESIAN_POINT('Ctrl Pts',(-410.866101565596,144.776338152558,-55.7617595366245)) ;
#3833=CARTESIAN_POINT('Ctrl Pts',(-410.879366221035,144.7870090043,-55.7411069784896)) ;
#3834=CARTESIAN_POINT('Ctrl Pts',(-410.915234441741,144.808141922543,-55.6850287041196)) ;
#3835=CARTESIAN_POINT('Ctrl Pts',(-410.940692427302,144.814359359455,-55.6449467921902)) ;
#3836=CARTESIAN_POINT('Ctrl Pts',(-410.977468137829,144.805890096303,-55.5875817150653)) ;
#3837=CARTESIAN_POINT('Ctrl Pts',(-410.989519327473,144.8002032316,-55.5688822109625)) ;
#3838=CARTESIAN_POINT('Ctrl Pts',(-411.012251139134,144.783206221826,-55.5339429555556)) ;
#3839=CARTESIAN_POINT('Ctrl Pts',(-411.022932248642,144.771897196056,-55.5177029769192)) ;
#3840=CARTESIAN_POINT('Ctrl Pts',(-411.042122001205,144.744713912751,-55.488934296626)) ;
#3841=CARTESIAN_POINT('Ctrl Pts',(-411.050872246538,144.728497413012,-55.4760433923461)) ;
#3842=CARTESIAN_POINT('Ctrl Pts',(-411.065896965649,144.692010331772,-55.454379230945)) ;
#3843=CARTESIAN_POINT('Ctrl Pts',(-411.072170663687,144.671739039288,-55.4456066332889)) ;
#3844=CARTESIAN_POINT('Ctrl Pts',(-411.086696644048,144.607536787114,-55.4260618107772)) ;
#3845=CARTESIAN_POINT('Ctrl Pts',(-411.090450063903,144.559939874016,-55.4223508921012)) ;
#3846=CARTESIAN_POINT('Ctrl Pts',(-411.088241395851,144.464267219023,-55.4288286532431)) ;
#3847=CARTESIAN_POINT('Ctrl Pts',(-411.080465387264,144.410212651786,-55.4418075470878)) ;
#3848=CARTESIAN_POINT('Ctrl Pts',(-411.053736123842,144.310165122957,-55.4820064660659)) ;
#3849=CARTESIAN_POINT('Ctrl Pts',(-411.034767278028,144.264167938495,-55.5092056101087)) ;
#3850=CARTESIAN_POINT('Ctrl Pts',(-410.994978355097,144.193112909149,-55.5644745189731)) ;
#3851=CARTESIAN_POINT('Ctrl Pts',(-410.971643135395,144.161135348259,-55.5962088184575)) ;
#3852=CARTESIAN_POINT('Ctrl Pts',(-410.945808745689,144.136110567136,-55.6308412032236)) ;
#3853=CARTESIAN_POINT('Ctrl Pts',(-410.945808745689,144.136110567136,-55.6308412032236)) ;
#3854=CARTESIAN_POINT('Ctrl Pts',(-410.945298830537,144.135616631912,-55.6315247718287)) ;
#3855=CARTESIAN_POINT('Ctrl Pts',(-410.944787948593,144.135125094846,-55.6322092502269)) ;
#3856=CARTESIAN_POINT('Ctrl Pts',(-410.917835749852,144.109399975703,-55.6683294231447)) ;
#3857=CARTESIAN_POINT('Ctrl Pts',(-410.888870545926,144.091437378252,-55.7066982382528)) ;
#3858=CARTESIAN_POINT('Ctrl Pts',(-410.840788144812,144.078228038009,-55.7709205875192)) ;
#3859=CARTESIAN_POINT('Ctrl Pts',(-410.818661134192,144.077445258792,-55.8006462833089)) ;
#3860=CARTESIAN_POINT('Ctrl Pts',(-410.777412893653,144.09142781431,-55.8574943436152)) ;
#3861=CARTESIAN_POINT('Ctrl Pts',(-410.758347903741,144.106361035004,-55.8846160834723)) ;
#3862=CARTESIAN_POINT('Ctrl Pts',(-410.728769308847,144.148260654197,-55.928959393124)) ;
#3863=CARTESIAN_POINT('Ctrl Pts',(-410.71704755088,144.176938464282,-55.947992188304)) ;
#3864=CARTESIAN_POINT('Ctrl Pts',(-410.702613810583,144.241832332789,-55.9746208221084)) ;
#3865=CARTESIAN_POINT('Ctrl Pts',(-410.699776826027,144.277977910514,-55.9823203715745)) ;
#3866=CARTESIAN_POINT('Ctrl Pts',(-410.700029842929,144.358940062948,-55.9898023477557)) ;
#3867=CARTESIAN_POINT('Ctrl Pts',(-410.705759375952,144.409817197619,-55.9862677279003)) ;
#3868=CARTESIAN_POINT('Ctrl Pts',(-410.725284786663,144.507540195539,-55.96540453293)) ;
#3869=CARTESIAN_POINT('Ctrl Pts',(-410.739117572465,144.554365057154,-55.9480121981902)) ;
#3870=CARTESIAN_POINT('Ctrl Pts',(-410.754250710349,144.59430346092,-55.9274355227232)) ;
#3871=CARTESIAN_POINT('Ctrl Pts',(-410.770827626794,144.638052192166,-55.9048957274367)) ;
#3872=CARTESIAN_POINT('Ctrl Pts',(-410.791856738387,144.681130902918,-55.874607897007)) ;
#3873=CARTESIAN_POINT('Ctrl Pts',(-410.827578363869,144.734108413478,-55.8209595835089)) ;
#3874=CARTESIAN_POINT('Ctrl Pts',(-410.840205301136,144.749908086438,-55.8016922908536)) ;
#3875=CARTESIAN_POINT('Ctrl Pts',(-410.853208211571,144.76317902685,-55.7816414442362)) ;
#3876=CARTESIAN_POINT('Origin',(-417.663667022248,147.594526517269,-60.2921051518733)) ;
#3877=CARTESIAN_POINT('',(-417.57694727224,147.778316277832,-60.071422101163)) ;
#3878=CARTESIAN_POINT('Origin',(-417.570614331253,148.427422997319,-56.3975416782406)) ;
#3879=CARTESIAN_POINT('',(-417.725577941508,148.178681425125,-56.3334019108612)) ;
#3880=CARTESIAN_POINT('Origin',(-440.720031578363,158.18696279177,-59.9690769391319)) ;
#3881=CARTESIAN_POINT('',(-438.755310766598,161.520385342634,-59.7481092393854)) ;
#3882=CARTESIAN_POINT('Origin',(-439.685550453976,159.855571466636,-60.3506446178581)) ;
#3883=CARTESIAN_POINT('',(-439.104150649365,160.896080139135,-59.9740600063125)) ;
#3884=CARTESIAN_POINT('Origin',(-439.685550453976,159.855571466636,-60.3506446178581)) ;
#3885=CARTESIAN_POINT('Origin',(-418.969932178152,146.01794126882,-57.8862684373746)) ;
#3886=CARTESIAN_POINT('',(-417.344023767738,148.808971130381,-57.5166886656118)) ;
#3887=CARTESIAN_POINT('Origin',(-418.2975194473,147.102536907483,-58.1342874285466)) ;
#3888=CARTESIAN_POINT('',(-417.692863650503,148.184665926884,-57.7426394325401)) ;
#3889=CARTESIAN_POINT('Origin',(-418.2975194473,147.102536907483,-58.1342874285466)) ;
#3890=CARTESIAN_POINT('Origin',(-428.991534950723,153.479054187111,-59.2424660232112)) ;
#3891=CARTESIAN_POINT('',(-420.601689255662,149.919110484244,-58.0440696072164)) ;
#3892=CARTESIAN_POINT('',(-421.811000864351,147.754852430924,-58.8273655362774)) ;
#3893=CARTESIAN_POINT('Origin',(-421.206345067555,148.836981450325,-58.4357175402709)) ;
#3894=CARTESIAN_POINT('Origin',(-421.206345067555,148.836981450325,-58.4357175402709)) ;
#3895=CARTESIAN_POINT('',(-428.386879153928,154.56118320651,-58.8508180272038)) ;
#3896=CARTESIAN_POINT('Ctrl Pts',(-421.81100086462,147.754852431096,-58.8273655363048)) ;
#3897=CARTESIAN_POINT('Ctrl Pts',(-421.853741332606,147.78033727655,-58.8317945622187)) ;
#3898=CARTESIAN_POINT('Ctrl Pts',(-421.896094847306,147.806514641693,-58.835972949529)) ;
#3899=CARTESIAN_POINT('Ctrl Pts',(-421.938043624344,147.833373922076,-58.8398988553431)) ;
#3900=CARTESIAN_POINT('Ctrl Pts',(-421.979570384227,147.860903662599,-58.8435707517313)) ;
#3901=CARTESIAN_POINT('Ctrl Pts',(-421.87615581497,147.692840521943,-58.5554346035487)) ;
#3902=CARTESIAN_POINT('Ctrl Pts',(-421.918896282955,147.718325367397,-58.5598636294598)) ;
#3903=CARTESIAN_POINT('Ctrl Pts',(-421.961208101147,147.744542417631,-58.5642160414727)) ;
#3904=CARTESIAN_POINT('Ctrl Pts',(-422.003073485147,147.771481068213,-58.5684899967742)) ;
#3905=CARTESIAN_POINT('Ctrl Pts',(-422.044475207505,147.799129814517,-58.5726837502117)) ;
#3906=CARTESIAN_POINT('Ctrl Pts',(-421.904621272866,147.696490374139,-58.2597391318533)) ;
#3907=CARTESIAN_POINT('Ctrl Pts',(-421.947361740345,147.721975220103,-58.2641681597162)) ;
#3908=CARTESIAN_POINT('Ctrl Pts',(-421.989655341618,147.748189934754,-58.2687098055672)) ;
#3909=CARTESIAN_POINT('Ctrl Pts',(-422.031484292327,147.775123913657,-58.2733622262356)) ;
#3910=CARTESIAN_POINT('Ctrl Pts',(-422.072831387722,147.80276565509,-58.2781234408005)) ;
#3911=CARTESIAN_POINT('Ctrl Pts',(-421.889780460918,147.772082270099,-57.9679944974231)) ;
#3912=CARTESIAN_POINT('Ctrl Pts',(-421.932520929689,147.797567114102,-57.9724235241036)) ;
#3913=CARTESIAN_POINT('Ctrl Pts',(-421.974824028932,147.823733452332,-57.9771518742023)) ;
#3914=CARTESIAN_POINT('Ctrl Pts',(-422.016671974219,147.850570680443,-57.9821777047032)) ;
#3915=CARTESIAN_POINT('Ctrl Pts',(-422.058047549007,147.878067356988,-57.9874988015613)) ;
#3916=CARTESIAN_POINT('Ctrl Pts',(-421.727691708573,148.170743063868,-57.2382494781475)) ;
#3917=CARTESIAN_POINT('Ctrl Pts',(-421.770432175108,148.196227912031,-57.2426785025898)) ;
#3918=CARTESIAN_POINT('Ctrl Pts',(-421.812839003795,148.22213912497,-57.2478738591303)) ;
#3919=CARTESIAN_POINT('Ctrl Pts',(-421.854894410256,148.248466098313,-57.2538337045393)) ;
#3920=CARTESIAN_POINT('Ctrl Pts',(-421.896581048473,148.275197708994,-57.260555242246)) ;
#3921=CARTESIAN_POINT('Ctrl Pts',(-421.300806933651,148.934613382335,-56.962373473136)) ;
#3922=CARTESIAN_POINT('Ctrl Pts',(-421.343547404315,148.960098222817,-56.9668025016983)) ;
#3923=CARTESIAN_POINT('Ctrl Pts',(-421.386227423225,148.985520587404,-56.9721744087365)) ;
#3924=CARTESIAN_POINT('Ctrl Pts',(-421.428829206111,149.010869871353,-56.9784873518901)) ;
#3925=CARTESIAN_POINT('Ctrl Pts',(-421.471335065955,149.036135561939,-56.9857383134319)) ;
#3926=CARTESIAN_POINT('Ctrl Pts',(-420.968923911373,149.464677297305,-57.115056870481)) ;
#3927=CARTESIAN_POINT('Ctrl Pts',(-421.011664377378,149.490162145958,-57.1194858972196)) ;
#3928=CARTESIAN_POINT('Ctrl Pts',(-421.054556786388,149.515245293827,-57.1247600927859)) ;
#3929=CARTESIAN_POINT('Ctrl Pts',(-421.09758335406,149.539916136489,-57.130877613928)) ;
#3930=CARTESIAN_POINT('Ctrl Pts',(-421.140726128437,149.564164584178,-57.1378355657362)) ;
#3931=CARTESIAN_POINT('Ctrl Pts',(-420.722334300366,149.804285292852,-57.5405450296813)) ;
#3932=CARTESIAN_POINT('Ctrl Pts',(-420.765074768969,149.829770137461,-57.5449740545007)) ;
#3933=CARTESIAN_POINT('Ctrl Pts',(-420.808124986228,149.854635948606,-57.5499759541758)) ;
#3934=CARTESIAN_POINT('Ctrl Pts',(-420.851467167597,149.878872122105,-57.5555488858895)) ;
#3935=CARTESIAN_POINT('Ctrl Pts',(-420.895083164411,149.90246883914,-57.5616902940697)) ;
#3936=CARTESIAN_POINT('Ctrl Pts',(-420.601689255787,149.919110484538,-58.0440696068916)) ;
#3937=CARTESIAN_POINT('Ctrl Pts',(-420.644429724086,149.944595329692,-58.0484986315046)) ;
#3938=CARTESIAN_POINT('Ctrl Pts',(-420.687557149156,149.969387657571,-58.0531782959234)) ;
#3939=CARTESIAN_POINT('Ctrl Pts',(-420.73105374647,149.993476863986,-58.0581067571802)) ;
#3940=CARTESIAN_POINT('Ctrl Pts',(-420.774901271003,150.016853221822,-58.0632818619355)) ;
#3941=CARTESIAN_POINT('',(-421.979570384495,147.860903662772,-58.8435707517587)) ;
#3942=CARTESIAN_POINT('',(-420.774901269911,150.016853221085,-58.0632818618408)) ;
#3943=CARTESIAN_POINT('Ctrl Pts',(-421.979570384227,147.860903662599,-58.8435707517313)) ;
#3944=CARTESIAN_POINT('Ctrl Pts',(-421.991728913092,147.849331654895,-58.7928258723717)) ;
#3945=CARTESIAN_POINT('Ctrl Pts',(-422.002346252811,147.84051778158,-58.7410831476083)) ;
#3946=CARTESIAN_POINT('Ctrl Pts',(-422.011341475327,147.834528590436,-58.6887406204753)) ;
#3947=CARTESIAN_POINT('Ctrl Pts',(-422.020433103031,147.828475210875,-58.6358371187712)) ;
#3948=CARTESIAN_POINT('Ctrl Pts',(-422.027867607628,147.825307398783,-58.5823212873917)) ;
#3949=CARTESIAN_POINT('Ctrl Pts',(-422.033587759229,147.825048295654,-58.5286122421676)) ;
#3950=CARTESIAN_POINT('Ctrl Pts',(-422.039326113949,147.824788367987,-58.4747322797561)) ;
#3951=CARTESIAN_POINT('Ctrl Pts',(-422.043339169569,147.827455647482,-58.4206582947106)) ;
#3952=CARTESIAN_POINT('Ctrl Pts',(-422.045595964448,147.833028188724,-58.366815344478)) ;
#3953=CARTESIAN_POINT('Ctrl Pts',(-422.047853400612,147.838602313442,-58.3129570943925)) ;
#3954=CARTESIAN_POINT('Ctrl Pts',(-422.048353573025,147.847083285091,-58.2593304370043)) ;
#3955=CARTESIAN_POINT('Ctrl Pts',(-422.047092431553,147.858404736773,-58.2063563350565)) ;
#3956=CARTESIAN_POINT('Ctrl Pts',(-422.045834620582,147.869696290064,-58.1535221304005)) ;
#3957=CARTESIAN_POINT('Ctrl Pts',(-422.042824794565,147.883813253942,-58.1013374569823)) ;
#3958=CARTESIAN_POINT('Ctrl Pts',(-422.038085680684,147.900646799821,-58.0502092009584)) ;
#3959=CARTESIAN_POINT('Ctrl Pts',(-422.033390570825,147.917324041432,-57.9995556853568)) ;
#3960=CARTESIAN_POINT('Ctrl Pts',(-422.026998175001,147.93666752218,-57.9499394416247)) ;
#3961=CARTESIAN_POINT('Ctrl Pts',(-422.018956495247,147.958530842599,-57.9017396362965)) ;
#3962=CARTESIAN_POINT('Ctrl Pts',(-422.010998890888,147.980165583,-57.8540437577363)) ;
#3963=CARTESIAN_POINT('Ctrl Pts',(-422.001426349376,148.004267619985,-57.8077352039805)) ;
#3964=CARTESIAN_POINT('Ctrl Pts',(-421.990310280786,148.030657100577,-57.7631597452683)) ;
#3965=CARTESIAN_POINT('Ctrl Pts',(-421.979286679813,148.056827063597,-57.718955081897)) ;
#3966=CARTESIAN_POINT('Ctrl Pts',(-421.966745154894,148.085246463539,-57.6764551336579)) ;
#3967=CARTESIAN_POINT('Ctrl Pts',(-421.952779447948,148.11570407895,-57.6359706624812)) ;
#3968=CARTESIAN_POINT('Ctrl Pts',(-421.940433622346,148.142628917739,-57.6001819822066)) ;
#3969=CARTESIAN_POINT('Ctrl Pts',(-421.926975175981,148.171146034768,-57.565968132908)) ;
#3970=CARTESIAN_POINT('Ctrl Pts',(-421.912484514256,148.201086851866,-57.5335232033393)) ;
#3971=CARTESIAN_POINT('Ctrl Pts',(-421.896469974511,148.234176328008,-57.4976662753414)) ;
#3972=CARTESIAN_POINT('Ctrl Pts',(-421.879196136062,148.269000982753,-57.4639750106296)) ;
#3973=CARTESIAN_POINT('Ctrl Pts',(-421.860784881679,148.305312756406,-57.4327011158411)) ;
#3974=CARTESIAN_POINT('Ctrl Pts',(-421.842112703721,148.34213913909,-57.4009840086437)) ;
#3975=CARTESIAN_POINT('Ctrl Pts',(-421.822270770487,148.380494869169,-57.3717533115999)) ;
#3976=CARTESIAN_POINT('Ctrl Pts',(-421.801403243559,148.42010078959,-57.3452246979226)) ;
#3977=CARTESIAN_POINT('Ctrl Pts',(-421.780249681462,148.460249595912,-57.3183324514799)) ;
#3978=CARTESIAN_POINT('Ctrl Pts',(-421.75804236051,148.501682853816,-57.2942169071462)) ;
#3979=CARTESIAN_POINT('Ctrl Pts',(-421.734946751139,148.544092520253,-57.2730543408166)) ;
#3980=CARTESIAN_POINT('Ctrl Pts',(-421.711554780111,148.587046385321,-57.2516202175384)) ;
#3981=CARTESIAN_POINT('Ctrl Pts',(-421.687251738192,148.631001603399,-57.2332153732183)) ;
#3982=CARTESIAN_POINT('Ctrl Pts',(-421.662222814826,148.675624522545,-57.2179731713502)) ;
#3983=CARTESIAN_POINT('Ctrl Pts',(-421.636685277877,148.721154225512,-57.2024212321921)) ;
#3984=CARTESIAN_POINT('Ctrl Pts',(-421.610392226587,148.767378743309,-57.1901618736898)) ;
#3985=CARTESIAN_POINT('Ctrl Pts',(-421.583551601739,148.813933965481,-57.1812842046049)) ;
#3986=CARTESIAN_POINT('Ctrl Pts',(-421.556710976892,148.860489187653,-57.17240653552)) ;
#3987=CARTESIAN_POINT('Ctrl Pts',(-421.529322989585,148.90737477357,-57.16691047875)) ;
#3988=CARTESIAN_POINT('Ctrl Pts',(-421.501603772458,148.95422189431,-57.1648332412647)) ;
#3989=CARTESIAN_POINT('Ctrl Pts',(-421.473633497548,149.001493317592,-57.1627371898772)) ;
#3990=CARTESIAN_POINT('Ctrl Pts',(-421.445326175544,149.048725223269,-57.1641221705782)) ;
#3991=CARTESIAN_POINT('Ctrl Pts',(-421.416909044811,149.095539089243,-57.1689740118675)) ;
#3992=CARTESIAN_POINT('Ctrl Pts',(-421.38842807649,149.142458120102,-57.1738367525629)) ;
#3993=CARTESIAN_POINT('Ctrl Pts',(-421.359837027396,149.188956868258,-57.1821818934184)) ;
#3994=CARTESIAN_POINT('Ctrl Pts',(-421.331366585001,149.234660067844,-57.1939432467292)) ;
#3995=CARTESIAN_POINT('Ctrl Pts',(-421.302964536217,149.28025347613,-57.205676346126)) ;
#3996=CARTESIAN_POINT('Ctrl Pts',(-421.274682736938,149.32505479751,-57.2208091745726)) ;
#3997=CARTESIAN_POINT('Ctrl Pts',(-421.246748794467,149.368702620244,-57.2392255460869)) ;
#3998=CARTESIAN_POINT('Ctrl Pts',(-421.218938200403,149.412157706508,-57.257560596101)) ;
#3999=CARTESIAN_POINT('Ctrl Pts',(-421.191472613444,149.454469114634,-57.2791501540304)) ;
#4000=CARTESIAN_POINT('Ctrl Pts',(-421.16457196597,149.495296490057,-57.3038309247386)) ;
#4001=CARTESIAN_POINT('Ctrl Pts',(-421.137930807612,149.535730036312,-57.3282736197127)) ;
#4002=CARTESIAN_POINT('Ctrl Pts',(-421.111843941636,149.574707731227,-57.3557480443583)) ;
#4003=CARTESIAN_POINT('Ctrl Pts',(-421.086517329051,149.611919830462,-57.3860495768582)) ;
#4004=CARTESIAN_POINT('Ctrl Pts',(-421.079319379369,149.622495694762,-57.3946614236062)) ;
#4005=CARTESIAN_POINT('Ctrl Pts',(-421.072182779199,149.632929093572,-57.403501342566)) ;
#4006=CARTESIAN_POINT('Ctrl Pts',(-421.065112107606,149.643213281796,-57.4125639715692)) ;
#4007=CARTESIAN_POINT('Ctrl Pts',(-421.040325659206,149.679264807793,-57.4443332855853)) ;
#4008=CARTESIAN_POINT('Ctrl Pts',(-421.01636439484,149.7134588299,-57.478823639632)) ;
#4009=CARTESIAN_POINT('Ctrl Pts',(-420.993412426575,149.74553265389,-57.5157706937358)) ;
#4010=CARTESIAN_POINT('Ctrl Pts',(-420.970680376631,149.777299156895,-57.5523637331431)) ;
#4011=CARTESIAN_POINT('Ctrl Pts',(-420.948938522522,149.806985666695,-57.591366512365)) ;
#4012=CARTESIAN_POINT('Ctrl Pts',(-420.928351251074,149.834367925265,-57.6324838549583)) ;
#4013=CARTESIAN_POINT('Ctrl Pts',(-420.907763979626,149.861750183835,-57.6736011975515)) ;
#4014=CARTESIAN_POINT('Ctrl Pts',(-420.888331463762,149.886827906802,-57.716833071087)) ;
#4015=CARTESIAN_POINT('Ctrl Pts',(-420.870201102755,149.909411860059,-57.7618467009588)) ;
#4016=CARTESIAN_POINT('Ctrl Pts',(-420.852668002297,149.931251840027,-57.8053774665191)) ;
#4017=CARTESIAN_POINT('Ctrl Pts',(-420.836352736448,149.950759582813,-57.8505743243232)) ;
#4018=CARTESIAN_POINT('Ctrl Pts',(-420.821371186243,149.967798922127,-57.8971032240582)) ;
#4019=CARTESIAN_POINT('Ctrl Pts',(-420.806644593601,149.98454828421,-57.9428402901869)) ;
#4020=CARTESIAN_POINT('Ctrl Pts',(-420.79320680203,149.998912402389,-57.989864350575)) ;
#4021=CARTESIAN_POINT('Ctrl Pts',(-420.781149569571,150.010797939994,-58.0378276646215)) ;
#4022=CARTESIAN_POINT('Ctrl Pts',(-420.779023792142,150.012893446376,-58.0462839443498)) ;
#4023=CARTESIAN_POINT('Ctrl Pts',(-420.776940879598,150.014912002863,-58.0547693444178)) ;
#4024=CARTESIAN_POINT('Ctrl Pts',(-420.774901271003,150.016853221822,-58.0632818619345)) ;
#4025=CARTESIAN_POINT('Origin',(-422.462167734146,146.589483527618,-59.2491443977063)) ;
#4026=CARTESIAN_POINT('Origin',(-419.950521499685,151.084480165857,-57.6222947862863)) ;
#4027=CARTESIAN_POINT('Ctrl Pts',(-420.601751328529,149.919051417961,-58.0438104715933)) ;
#4028=CARTESIAN_POINT('Ctrl Pts',(-420.644495899909,149.944538709794,-58.0482399216921)) ;
#4029=CARTESIAN_POINT('Ctrl Pts',(-420.687627462681,149.969333389136,-58.0529202253984)) ;
#4030=CARTESIAN_POINT('Ctrl Pts',(-420.731128227209,149.993424848719,-58.0578495392067)) ;
#4031=CARTESIAN_POINT('Ctrl Pts',(-420.774979943197,150.016803358696,-58.0630257089282)) ;
#4032=CARTESIAN_POINT('Ctrl Pts',(-420.49059208657,150.024888462511,-58.5075145316237)) ;
#4033=CARTESIAN_POINT('Ctrl Pts',(-420.533336657653,150.050375754802,-58.5119439819544)) ;
#4034=CARTESIAN_POINT('Ctrl Pts',(-420.576539371367,150.075102689897,-58.5163274770719)) ;
#4035=CARTESIAN_POINT('Ctrl Pts',(-420.620182438101,150.099058660511,-58.5206631733476)) ;
#4036=CARTESIAN_POINT('Ctrl Pts',(-420.664247518745,150.122234021346,-58.5249492871398)) ;
#4037=CARTESIAN_POINT('Ctrl Pts',(-420.485369825263,149.940704294701,-59.0423098699552)) ;
#4038=CARTESIAN_POINT('Ctrl Pts',(-420.528114397322,149.966191584884,-59.0467393230098)) ;
#4039=CARTESIAN_POINT('Ctrl Pts',(-420.571320454056,149.990972404078,-59.0507805059011)) ;
#4040=CARTESIAN_POINT('Ctrl Pts',(-420.61497020581,150.015036144952,-59.0544315754972)) ;
#4041=CARTESIAN_POINT('Ctrl Pts',(-420.659045309316,150.038373095001,-59.0576911748749)) ;
#4042=CARTESIAN_POINT('Ctrl Pts',(-420.6241938334,149.627915888419,-59.5024474146452)) ;
#4043=CARTESIAN_POINT('Ctrl Pts',(-420.666938401923,149.653403185214,-59.5068768636633)) ;
#4044=CARTESIAN_POINT('Ctrl Pts',(-420.710055598583,149.678384217066,-59.5106235194951)) ;
#4045=CARTESIAN_POINT('Ctrl Pts',(-420.753527634076,149.702848376139,-59.513685538623)) ;
#4046=CARTESIAN_POINT('Ctrl Pts',(-420.797336275705,149.726785700566,-59.5160619320858)) ;
#4047=CARTESIAN_POINT('Ctrl Pts',(-421.013789367829,148.908194055108,-59.884135012707)) ;
#4048=CARTESIAN_POINT('Ctrl Pts',(-421.056533940723,148.933681343997,-59.8885644652487)) ;
#4049=CARTESIAN_POINT('Ctrl Pts',(-421.09940176579,148.959123054161,-59.8920668107065)) ;
#4050=CARTESIAN_POINT('Ctrl Pts',(-421.142375053396,148.984508578293,-59.8946402059013)) ;
#4051=CARTESIAN_POINT('Ctrl Pts',(-421.185435882405,149.009827379056,-59.8962839664587)) ;
#4052=CARTESIAN_POINT('Ctrl Pts',(-421.451996513475,148.217919515022,-59.627275259948)) ;
#4053=CARTESIAN_POINT('Ctrl Pts',(-421.49474108344,148.243406809216,-59.6317047101229)) ;
#4054=CARTESIAN_POINT('Ctrl Pts',(-421.537328418939,148.269290353584,-59.6353714662152)) ;
#4055=CARTESIAN_POINT('Ctrl Pts',(-421.579740730352,148.295559540816,-59.63827368484)) ;
#4056=CARTESIAN_POINT('Ctrl Pts',(-421.621960446587,148.322203282162,-59.6404104766189)) ;
#4057=CARTESIAN_POINT('Ctrl Pts',(-421.613231704278,147.983523447751,-59.4200694389356)) ;
#4058=CARTESIAN_POINT('Ctrl Pts',(-421.655976274758,148.00901074047,-59.4244988926215)) ;
#4059=CARTESIAN_POINT('Ctrl Pts',(-421.698460406657,148.035044317106,-59.4282982785714)) ;
#4060=CARTESIAN_POINT('Ctrl Pts',(-421.740666310351,148.061613570312,-59.4314657535976)) ;
#4061=CARTESIAN_POINT('Ctrl Pts',(-421.782576543553,148.088707224125,-59.4340002626073)) ;
#4062=CARTESIAN_POINT('Ctrl Pts',(-421.736314996746,147.825908589189,-59.1392295361033)) ;
#4063=CARTESIAN_POINT('Ctrl Pts',(-421.779059567893,147.851395881237,-59.1436589872169)) ;
#4064=CARTESIAN_POINT('Ctrl Pts',(-421.821464916546,147.87753034417,-59.1476381330355)) ;
#4065=CARTESIAN_POINT('Ctrl Pts',(-421.863513253218,147.904301370467,-59.1511651300512)) ;
#4066=CARTESIAN_POINT('Ctrl Pts',(-421.905187233809,147.931697558431,-59.1542386991413)) ;
#4067=CARTESIAN_POINT('Ctrl Pts',(-421.811062973951,147.754793329066,-58.8271062522543)) ;
#4068=CARTESIAN_POINT('Ctrl Pts',(-421.8538075451,147.780280621111,-58.8315357033629)) ;
#4069=CARTESIAN_POINT('Ctrl Pts',(-421.89616504891,147.806460603649,-58.835714633705)) ;
#4070=CARTESIAN_POINT('Ctrl Pts',(-421.938117695878,147.833322669176,-58.8396411998575)) ;
#4071=CARTESIAN_POINT('Ctrl Pts',(-421.979648201636,147.860855359163,-58.8433138732736)) ;
#4072=CARTESIAN_POINT('Origin',(-421.377235834177,148.938878434349,-58.4534262754551)) ;
#4073=CARTESIAN_POINT('Origin',(-428.991534950723,153.479054187111,-59.2424660232112)) ;
#4074=CARTESIAN_POINT('',(-423.25286169586,147.847682592174,-57.9134552983687)) ;
#4075=CARTESIAN_POINT('',(-421.302624061803,151.113877299569,-57.939556238929)) ;
#4076=CARTESIAN_POINT('Origin',(-422.232863749181,149.44906342357,-58.542091617402)) ;
#4077=CARTESIAN_POINT('',(-428.061295263345,155.143868063109,-58.6399306447382)) ;
#4078=CARTESIAN_POINT('Origin',(-422.232863749181,149.44906342357,-58.542091617402)) ;
#4079=CARTESIAN_POINT('Origin',(-422.232863749181,149.44906342357,-58.542091617402)) ;
#4080=CARTESIAN_POINT('',(-421.129412046089,151.016134561919,-57.9203439835838)) ;
#4081=CARTESIAN_POINT('',(-423.084516151496,147.741789646215,-57.8941779127654)) ;
#4082=CARTESIAN_POINT('Origin',(-422.061972981251,149.347166438823,-58.5243828819896)) ;
#4083=CARTESIAN_POINT('Origin',(-425.292857589218,144.644920929381,-56.6561826603022)) ;
#4084=CARTESIAN_POINT('Origin',(-422.061972981251,149.347166438823,-58.5243828819896)) ;
#4085=CARTESIAN_POINT('Origin',(-428.991534950723,153.479054187111,-59.2424660232112)) ;
#4086=CARTESIAN_POINT('',(-420.236817124951,150.533858084077,-57.816462643087)) ;
#4087=CARTESIAN_POINT('',(-428.038039271161,155.185488410009,-58.6248672602764)) ;
#4088=CARTESIAN_POINT('',(-422.143809736987,147.120988422025,-59.0516550729336)) ;
#4089=CARTESIAN_POINT('Origin',(-421.190314057423,148.827422644927,-58.4340563099994)) ;
#4090=CARTESIAN_POINT('Origin',(-421.190314057423,148.827422644927,-58.4340563099994)) ;
#4091=CARTESIAN_POINT('Origin',(-422.147365028502,149.39808312813,-58.5332317226227)) ;
#4092=CARTESIAN_POINT('',(-422.343986042163,147.246924259843,-59.0708987663161)) ;
#4093=CARTESIAN_POINT('',(-420.442506399576,150.649927582747,-57.8392771818555)) ;
#4094=CARTESIAN_POINT('Origin',(-421.393246844343,148.948425314316,-58.4550854333019)) ;
#4095=CARTESIAN_POINT('Origin',(-421.393246844343,148.948425314316,-58.4550854333019)) ;
#4096=CARTESIAN_POINT('',(-421.217125341124,151.062897004128,-57.9306963441498)) ;
#4097=CARTESIAN_POINT('Ctrl Pts',(-420.442317319748,150.650212478691,-57.8403702955082)) ;
#4098=CARTESIAN_POINT('Ctrl Pts',(-420.390229898959,150.622444850762,-57.8342240564197)) ;
#4099=CARTESIAN_POINT('Ctrl Pts',(-420.338559599104,150.593830011908,-57.8283703755451)) ;
#4100=CARTESIAN_POINT('Ctrl Pts',(-420.287328108581,150.564379524318,-57.8228118120409)) ;
#4101=CARTESIAN_POINT('Ctrl Pts',(-420.236556568021,150.534105993319,-57.8175505566696)) ;
#4102=CARTESIAN_POINT('Ctrl Pts',(-420.626777418833,150.474826238209,-57.069496565559)) ;
#4103=CARTESIAN_POINT('Ctrl Pts',(-420.574957527116,150.446804241574,-57.0622322995815)) ;
#4104=CARTESIAN_POINT('Ctrl Pts',(-420.523465654325,150.418019752801,-57.0556329570686)) ;
#4105=CARTESIAN_POINT('Ctrl Pts',(-420.472323377486,150.388484440006,-57.049701562745)) ;
#4106=CARTESIAN_POINT('Ctrl Pts',(-420.42155183722,150.358210908514,-57.0444403073611)) ;
#4107=CARTESIAN_POINT('Ctrl Pts',(-420.998424490206,149.96520818523,-56.4154402406386)) ;
#4108=CARTESIAN_POINT('Ctrl Pts',(-420.94714361401,149.936447067719,-56.4072273700832)) ;
#4109=CARTESIAN_POINT('Ctrl Pts',(-420.896011233862,149.907169627505,-56.3999953620422)) ;
#4110=CARTESIAN_POINT('Ctrl Pts',(-420.845048702436,149.877387840324,-56.3937476359878)) ;
#4111=CARTESIAN_POINT('Ctrl Pts',(-420.794277160261,149.847114311642,-56.3884863828677)) ;
#4112=CARTESIAN_POINT('Ctrl Pts',(-421.500791590854,149.167595269917,-56.1570621835743)) ;
#4113=CARTESIAN_POINT('Ctrl Pts',(-421.450239313169,149.137677350129,-56.1484745773338)) ;
#4114=CARTESIAN_POINT('Ctrl Pts',(-421.399592868659,149.107628385508,-56.1409926414793)) ;
#4115=CARTESIAN_POINT('Ctrl Pts',(-421.348873306703,149.077460833301,-56.1346199518746)) ;
#4116=CARTESIAN_POINT('Ctrl Pts',(-421.298101767752,149.047187299145,-56.129358699136)) ;
#4117=CARTESIAN_POINT('Ctrl Pts',(-422.182013907982,147.96033734627,-56.529835127009)) ;
#4118=CARTESIAN_POINT('Ctrl Pts',(-422.132449635391,147.928668489913,-56.5217881696355)) ;
#4119=CARTESIAN_POINT('Ctrl Pts',(-422.082462134238,147.897451749959,-56.5146668157615)) ;
#4120=CARTESIAN_POINT('Ctrl Pts',(-422.032072042464,147.866700312821,-56.5084744157967)) ;
#4121=CARTESIAN_POINT('Ctrl Pts',(-421.981300500553,147.836426784044,-56.5032131606753)) ;
#4122=CARTESIAN_POINT('Ctrl Pts',(-422.464086691705,147.292074351448,-57.6530293612976)) ;
#4123=CARTESIAN_POINT('Ctrl Pts',(-422.414931518073,147.259436291465,-57.6466114130534)) ;
#4124=CARTESIAN_POINT('Ctrl Pts',(-422.365216863686,147.227573145683,-57.640576517863)) ;
#4125=CARTESIAN_POINT('Ctrl Pts',(-422.314963196154,147.196498504072,-57.6349273479934)) ;
#4126=CARTESIAN_POINT('Ctrl Pts',(-422.264191655957,147.166224972182,-57.6296660942382)) ;
#4127=CARTESIAN_POINT('Ctrl Pts',(-422.49553424485,147.155810241822,-58.1336286388597)) ;
#4128=CARTESIAN_POINT('Ctrl Pts',(-422.446424681794,147.122974551427,-58.127907720542)) ;
#4129=CARTESIAN_POINT('Ctrl Pts',(-422.396740446769,147.090979597685,-58.1223377058509)) ;
#4130=CARTESIAN_POINT('Ctrl Pts',(-422.346501988429,147.059839052819,-58.1169209767701)) ;
#4131=CARTESIAN_POINT('Ctrl Pts',(-422.295730447237,147.029565522422,-58.1116597241416)) ;
#4132=CARTESIAN_POINT('Ctrl Pts',(-422.451413471441,147.144684274654,-58.623417159732)) ;
#4133=CARTESIAN_POINT('Ctrl Pts',(-422.402239917998,147.111832448195,-58.6184066016194)) ;
#4134=CARTESIAN_POINT('Ctrl Pts',(-422.352513005096,147.079826732491,-58.613310356972)) ;
#4135=CARTESIAN_POINT('Ctrl Pts',(-422.302253207981,147.048680806466,-58.6081305121877)) ;
#4136=CARTESIAN_POINT('Ctrl Pts',(-422.251481667166,147.018407275726,-58.6028692579116)) ;
#4137=CARTESIAN_POINT('Ctrl Pts',(-422.343792618447,147.247216634306,-59.0719908009918)) ;
#4138=CARTESIAN_POINT('Ctrl Pts',(-422.294462978472,147.214513514342,-59.0676308259597)) ;
#4139=CARTESIAN_POINT('Ctrl Pts',(-422.244631964546,147.182606977597,-59.0629684839705)) ;
#4140=CARTESIAN_POINT('Ctrl Pts',(-422.194320116926,147.151510641041,-59.0580055905041)) ;
#4141=CARTESIAN_POINT('Ctrl Pts',(-422.143548576108,147.121237110302,-59.0527443362252)) ;
#4142=CARTESIAN_POINT('Origin',(-422.446249450215,146.579713262273,-59.2475425158174)) ;
#4143=CARTESIAN_POINT('Origin',(-419.934490494852,151.074921350906,-57.6206335614338)) ;
#4144=CARTESIAN_POINT('Ctrl Pts',(-422.34418631909,147.246799897813,-59.070237373874)) ;
#4145=CARTESIAN_POINT('Ctrl Pts',(-422.294863584558,147.214100818998,-59.0658753144168)) ;
#4146=CARTESIAN_POINT('Ctrl Pts',(-422.245039410828,147.182198310169,-59.0612118137456)) ;
#4147=CARTESIAN_POINT('Ctrl Pts',(-422.194734329872,147.151105983027,-59.0562486877295)) ;
#4148=CARTESIAN_POINT('Ctrl Pts',(-422.143969473837,147.120836438223,-59.0509881261684)) ;
#4149=CARTESIAN_POINT('Ctrl Pts',(-422.228145324003,147.357174965478,-59.554938735971)) ;
#4150=CARTESIAN_POINT('Ctrl Pts',(-422.178654335311,147.324635925487,-59.5512794714222)) ;
#4151=CARTESIAN_POINT('Ctrl Pts',(-422.128717945445,147.292840153624,-59.5470846957269)) ;
#4152=CARTESIAN_POINT('Ctrl Pts',(-422.078356756426,147.261801194959,-59.5423559321871)) ;
#4153=CARTESIAN_POINT('Ctrl Pts',(-422.027591900393,147.231531650153,-59.5370953706258)) ;
#4154=CARTESIAN_POINT('Ctrl Pts',(-422.037973303002,147.600208882302,-59.9916847370896)) ;
#4155=CARTESIAN_POINT('Ctrl Pts',(-421.98820657396,147.56802223003,-59.9886587324345)) ;
#4156=CARTESIAN_POINT('Ctrl Pts',(-421.938086280561,147.536461481207,-59.9848863063301)) ;
#4157=CARTESIAN_POINT('Ctrl Pts',(-421.88763313952,147.505540034306,-59.9803687186285)) ;
#4158=CARTESIAN_POINT('Ctrl Pts',(-421.836868283048,147.475270489885,-59.9751081589749)) ;
#4159=CARTESIAN_POINT('Ctrl Pts',(-421.789025698594,147.961261985461,-60.3165314648779)) ;
#4160=CARTESIAN_POINT('Ctrl Pts',(-421.738898007252,147.92959884269,-60.3139764756352)) ;
#4161=CARTESIAN_POINT('Ctrl Pts',(-421.688536972012,147.898387245812,-60.310518189728)) ;
#4162=CARTESIAN_POINT('Ctrl Pts',(-421.637963459867,147.867640375442,-60.3061576708561)) ;
#4163=CARTESIAN_POINT('Ctrl Pts',(-421.587198603022,147.837370832091,-60.3008971087469)) ;
#4164=CARTESIAN_POINT('Ctrl Pts',(-421.102314662438,149.040189908199,-60.7351426238331)) ;
#4165=CARTESIAN_POINT('Ctrl Pts',(-421.051191269308,149.010091165465,-60.7331946003715)) ;
#4166=CARTESIAN_POINT('Ctrl Pts',(-421.000166157263,148.97992293485,-60.7301411271694)) ;
#4167=CARTESIAN_POINT('Ctrl Pts',(-420.94926060771,148.949697745786,-60.7259830153771)) ;
#4168=CARTESIAN_POINT('Ctrl Pts',(-420.898495752919,148.919428198737,-60.7207224546085)) ;
#4169=CARTESIAN_POINT('Ctrl Pts',(-420.483542510817,150.179465060839,-60.1508967990536)) ;
#4170=CARTESIAN_POINT('Ctrl Pts',(-420.431521929361,150.151018209618,-60.1481016477795)) ;
#4171=CARTESIAN_POINT('Ctrl Pts',(-420.379898441695,150.121951700366,-60.1444831869925)) ;
#4172=CARTESIAN_POINT('Ctrl Pts',(-420.328693702851,150.092277374683,-60.1400425803007)) ;
#4173=CARTESIAN_POINT('Ctrl Pts',(-420.27792884495,150.062007833199,-60.1347820175111)) ;
#4174=CARTESIAN_POINT('Ctrl Pts',(-420.259174590128,150.682575177394,-59.4211440937216)) ;
#4175=CARTESIAN_POINT('Ctrl Pts',(-420.206828682934,150.654857817706,-59.4172908307359)) ;
#4176=CARTESIAN_POINT('Ctrl Pts',(-420.154988222027,150.626277836902,-59.4129666696233)) ;
#4177=CARTESIAN_POINT('Ctrl Pts',(-420.103674997724,150.596846773186,-59.4081732146125)) ;
#4178=CARTESIAN_POINT('Ctrl Pts',(-420.052910142311,150.566577226921,-59.4029126553418)) ;
#4179=CARTESIAN_POINT('Ctrl Pts',(-420.266515670992,150.817595489973,-58.5733881509068)) ;
#4180=CARTESIAN_POINT('Ctrl Pts',(-420.214180408597,150.790073902018,-58.5683056838671)) ;
#4181=CARTESIAN_POINT('Ctrl Pts',(-420.162347047,150.761624490549,-58.5631617112019)) ;
#4182=CARTESIAN_POINT('Ctrl Pts',(-420.111037372064,150.732258712297,-58.5579583485471)) ;
#4183=CARTESIAN_POINT('Ctrl Pts',(-420.060272516065,150.701989167613,-58.5526977858246)) ;
#4184=CARTESIAN_POINT('Ctrl Pts',(-420.442710151574,150.649797874219,-57.8386129852327)) ;
#4185=CARTESIAN_POINT('Ctrl Pts',(-420.390630362941,150.622032987744,-57.8324651274969)) ;
#4186=CARTESIAN_POINT('Ctrl Pts',(-420.33896738815,150.593421309605,-57.8266105987488)) ;
#4187=CARTESIAN_POINT('Ctrl Pts',(-420.287742906723,150.563974397833,-57.8210519581525)) ;
#4188=CARTESIAN_POINT('Ctrl Pts',(-420.236978050927,150.533704852778,-57.8157913956035)) ;
#4189=CARTESIAN_POINT('Origin',(-428.991534950723,153.479054187111,-59.2424660232112)) ;
#4190=CARTESIAN_POINT('',(-421.667494954702,150.499130901467,-58.167168236128)) ;
#4191=CARTESIAN_POINT('',(-428.410135146112,154.51956285961,-58.8658814116656)) ;
#4192=CARTESIAN_POINT('Origin',(-422.248894759313,149.458622228968,-58.5437528476736)) ;
#4193=CARTESIAN_POINT('Origin',(-422.147365028502,149.39808312813,-58.5332317226227)) ;
#4194=CARTESIAN_POINT('',(-421.461805686039,150.383061400504,-58.1443536829051)) ;
#4195=CARTESIAN_POINT('Origin',(-422.045961972393,149.337619559579,-58.522723724371)) ;
#4196=CARTESIAN_POINT('',(-421.565965223891,150.438591800629,-58.1566471110771)) ;
#4197=CARTESIAN_POINT('Origin',(-422.248894759313,149.458622228968,-58.5437528476736)) ;
#4198=CARTESIAN_POINT('Origin',(-419.45817569718,154.453063856963,-56.7361467122547)) ;
#4296=UNCERTAINTY_MEASURE_WITH_UNIT(LENGTH_MEASURE(0.01),#4305,
'DISTANCE_ACCURACY_VALUE',
'Maximum model space distance between geometric entities at asserted c
onnectivities') ;
#4298=UNCERTAINTY_MEASURE_WITH_UNIT(LENGTH_MEASURE(0.01),#4305,
'DISTANCE_ACCURACY_VALUE',
'Maximum model space distance between geometric entities at asserted c
onnectivities') ;
#4302=(
GEOMETRIC_REPRESENTATION_CONTEXT(3)
GLOBAL_UNCERTAINTY_ASSIGNED_CONTEXT((#4296))
GLOBAL_UNIT_ASSIGNED_CONTEXT((#4305,#4307,#4308))
REPRESENTATION_CONTEXT('','3D')
) ;
#4304=(
GEOMETRIC_REPRESENTATION_CONTEXT(3)
GLOBAL_UNCERTAINTY_ASSIGNED_CONTEXT((#4298))
GLOBAL_UNIT_ASSIGNED_CONTEXT((#4305,#4307,#4308))
REPRESENTATION_CONTEXT('','3D')
) ;
#4305=(
LENGTH_UNIT()
NAMED_UNIT(*)
SI_UNIT(.MILLI.,.METRE.)
) ;
#4307=(
NAMED_UNIT(*)
PLANE_ANGLE_UNIT()
SI_UNIT($,.RADIAN.)
) ;
#4308=(
NAMED_UNIT(*)
SI_UNIT($,.STERADIAN.)
SOLID_ANGLE_UNIT()
) ;
#4312=SHAPE_DEFINITION_REPRESENTATION(#4317,#4333) ;
#4317=PRODUCT_DEFINITION_SHAPE('',$,#4339) ;
#4333=SHAPE_REPRESENTATION('',(#2366),#4302) ;
#4335=PRODUCT_DEFINITION_CONTEXT('part definition',#4352,'design') ;
#4339=PRODUCT_DEFINITION('Nozzle','Nozzle',#4344,#4335) ;
#4344=PRODUCT_DEFINITION_FORMATION('',$,#4357) ;
#4352=APPLICATION_CONTEXT(
'Core Data for Automotive Mechanical Design Process') ;
#4353=PRODUCT_CONTEXT('part definition',#4352,'mechanical') ;
#4357=PRODUCT('Nozzle','Nozzle',$,(#4353)) ;
#4360=PRESENTATION_STYLE_ASSIGNMENT((#4364)) ;
#4361=PRESENTATION_STYLE_ASSIGNMENT((#4365)) ;
#4364=SURFACE_STYLE_USAGE(.BOTH.,#4368) ;
#4365=SURFACE_STYLE_USAGE(.BOTH.,#4369) ;
#4368=SURFACE_SIDE_STYLE('',(#4372)) ;
#4369=SURFACE_SIDE_STYLE('',(#4373)) ;
#4372=SURFACE_STYLE_FILL_AREA(#4376) ;
#4373=SURFACE_STYLE_FILL_AREA(#4377) ;
#4376=FILL_AREA_STYLE('Opaque(243,203,124)',(#4380)) ;
#4377=FILL_AREA_STYLE('Opaque(210,210,255)',(#4381)) ;
#4380=FILL_AREA_STYLE_COLOUR('Opaque(243,203,124)',#4384) ;
#4381=FILL_AREA_STYLE_COLOUR('Opaque(210,210,255)',#4385) ;
#4384=COLOUR_RGB('Opaque(243,203,124)', 0.09019608, 0.27058824, 0.51372549) ;
#4385=COLOUR_RGB('Opaque(210,210,255)', 0.72549020, 0.75294118, 0.79215686) ;
ENDSEC;
END-ISO-10303-21;
